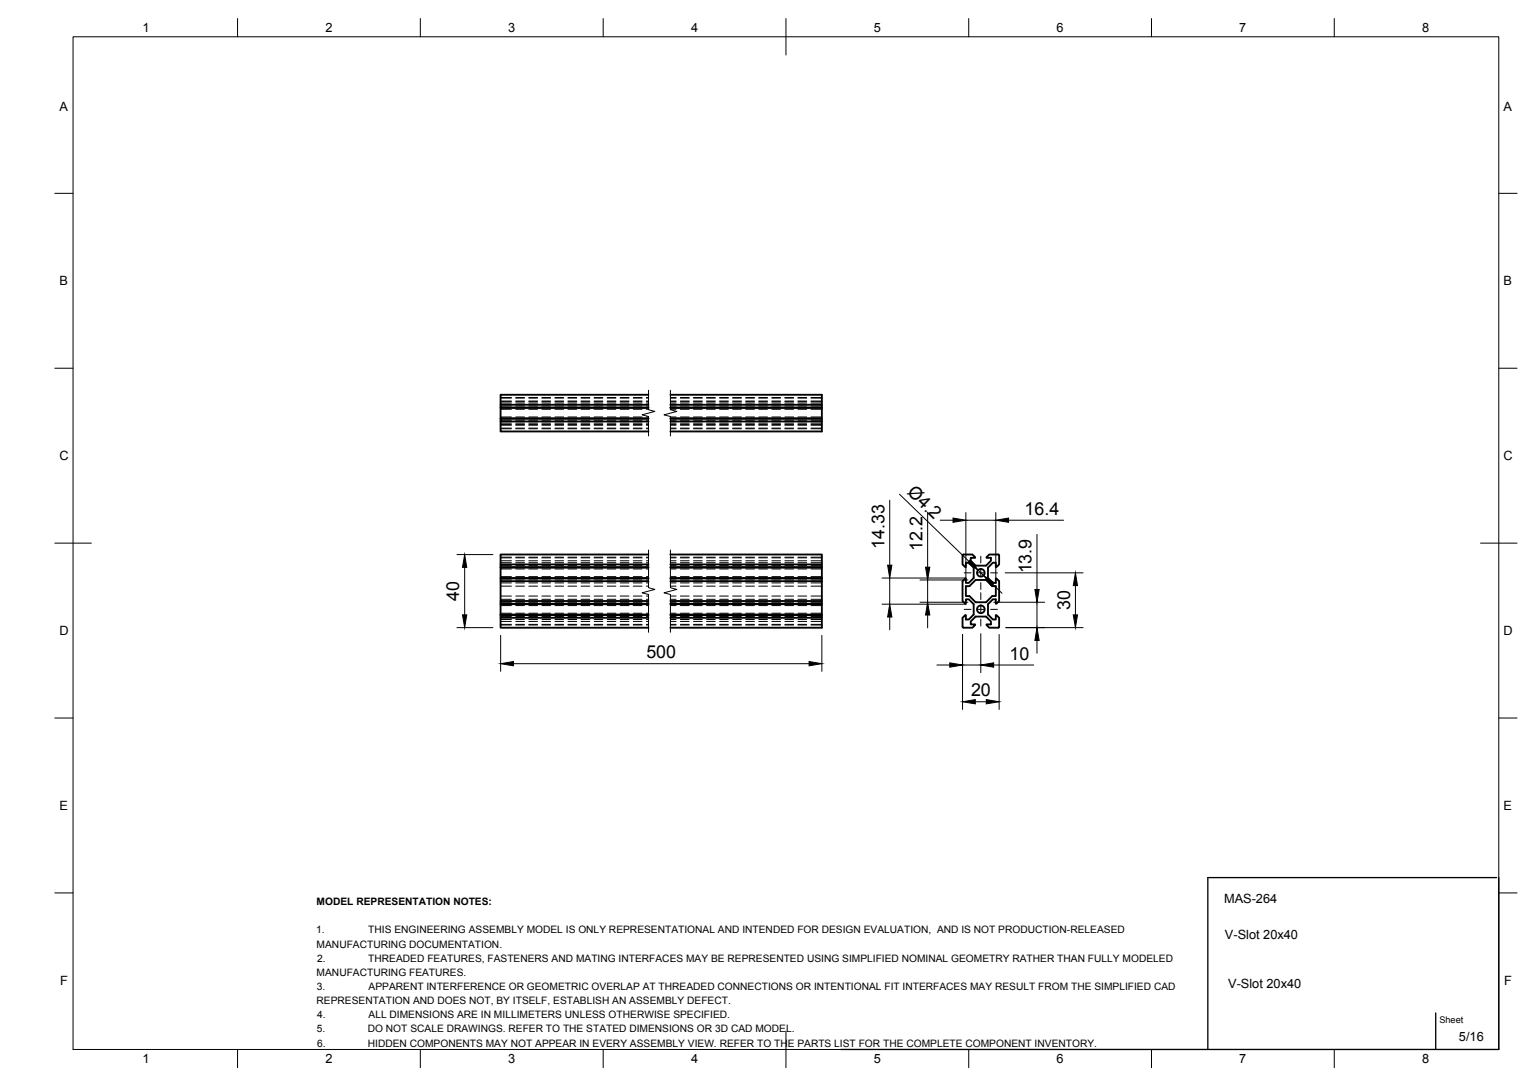
ISO-10303-21;
HEADER;
/* Generated by software containing ST-Developer
 * from STEP Tools, Inc. (www.steptools.com) 
 */

FILE_DESCRIPTION(
/* description */ (''),
/* implementation_level */ '2;1');

FILE_NAME(
/* name */ 'V-Slot 20x40.step',
/* time_stamp */ '2026-10-12T15:37:13-07:00',
/* author */ (''),
/* organization */ (''),
/* preprocessor_version */ 'ST-DEVELOPER v20.2',
/* originating_system */ 'Autodesk Translation Framework v15.15.0.0',
/* authorisation */ '');

FILE_SCHEMA (('AUTOMOTIVE_DESIGN { 1 0 10303 214 3 1 1 }'));
ENDSEC;

DATA;
#10=MECHANICAL_DESIGN_GEOMETRIC_PRESENTATION_REPRESENTATION('',(#350),#36460);
#111=SHAPE_REPRESENTATION_RELATIONSHIP('SRR','None',#36523,#124);
#124=ADVANCED_BREP_SHAPE_REPRESENTATION('',(#382),#36452);
#172=FACE_BOUND('',#2091,.T.);
#173=FACE_BOUND('',#2092,.T.);
#174=FACE_BOUND('',#2093,.T.);
#175=FACE_BOUND('',#2142,.T.);
#176=FACE_BOUND('',#2143,.T.);
#177=FACE_BOUND('',#2144,.T.);
#350=STYLED_ITEM('',(#36598),#382);
#382=MANIFOLD_SOLID_BREP('Body1',#11286);
#540=PLANE('',#12010);
#541=PLANE('',#12011);
#542=PLANE('',#12012);
#543=PLANE('',#12013);
#544=PLANE('',#12014);
#545=PLANE('',#12018);
#546=PLANE('',#12019);
#547=PLANE('',#12020);
#548=PLANE('',#12021);
#549=PLANE('',#12022);
#550=PLANE('',#12023);
#551=PLANE('',#12024);
#552=PLANE('',#12025);
#553=PLANE('',#12026);
#554=PLANE('',#12030);
#555=PLANE('',#12031);
#556=PLANE('',#12032);
#557=PLANE('',#12033);
#558=PLANE('',#12034);
#559=PLANE('',#12035);
#560=PLANE('',#12036);
#561=PLANE('',#12037);
#562=PLANE('',#12038);
#563=PLANE('',#12039);
#564=PLANE('',#12040);
#565=PLANE('',#12041);
#566=PLANE('',#12042);
#567=PLANE('',#12043);
#568=PLANE('',#12044);
#569=PLANE('',#12045);
#570=PLANE('',#12046);
#571=PLANE('',#12047);
#572=PLANE('',#12051);
#573=PLANE('',#12052);
#574=PLANE('',#12053);
#575=PLANE('',#12054);
#576=PLANE('',#12055);
#577=PLANE('',#12056);
#578=PLANE('',#12057);
#579=PLANE('',#12058);
#580=PLANE('',#12059);
#581=PLANE('',#12060);
#582=PLANE('',#12061);
#583=PLANE('',#12062);
#584=PLANE('',#12063);
#585=PLANE('',#12067);
#586=PLANE('',#12068);
#587=PLANE('',#12069);
#588=PLANE('',#12070);
#589=PLANE('',#12071);
#590=PLANE('',#12074);
#591=PLANE('',#12075);
#592=PLANE('',#12076);
#593=PLANE('',#12077);
#594=PLANE('',#12078);
#595=PLANE('',#12079);
#596=PLANE('',#12080);
#597=PLANE('',#12081);
#598=PLANE('',#12082);
#599=PLANE('',#12085);
#600=PLANE('',#12086);
#601=PLANE('',#12087);
#602=PLANE('',#12088);
#603=PLANE('',#12089);
#604=PLANE('',#12090);
#605=PLANE('',#12091);
#606=PLANE('',#12092);
#607=PLANE('',#12093);
#608=PLANE('',#12094);
#609=PLANE('',#12095);
#610=PLANE('',#12096);
#611=PLANE('',#12097);
#612=PLANE('',#12098);
#613=PLANE('',#12099);
#614=PLANE('',#12100);
#615=PLANE('',#12101);
#616=PLANE('',#12102);
#617=PLANE('',#12103);
#618=PLANE('',#12106);
#619=PLANE('',#12107);
#620=PLANE('',#12108);
#621=PLANE('',#12109);
#622=PLANE('',#12110);
#623=PLANE('',#12111);
#624=PLANE('',#12112);
#625=PLANE('',#12113);
#626=PLANE('',#12114);
#627=PLANE('',#12115);
#628=PLANE('',#12116);
#629=PLANE('',#12117);
#1389=FACE_OUTER_BOUND('',#2043,.T.);
#1390=FACE_OUTER_BOUND('',#2044,.T.);
#1391=FACE_OUTER_BOUND('',#2045,.T.);
#1392=FACE_OUTER_BOUND('',#2046,.T.);
#1393=FACE_OUTER_BOUND('',#2047,.T.);
#1394=FACE_OUTER_BOUND('',#2048,.T.);
#1395=FACE_OUTER_BOUND('',#2049,.T.);
#1396=FACE_OUTER_BOUND('',#2050,.T.);
#1397=FACE_OUTER_BOUND('',#2051,.T.);
#1398=FACE_OUTER_BOUND('',#2052,.T.);
#1399=FACE_OUTER_BOUND('',#2053,.T.);
#1400=FACE_OUTER_BOUND('',#2054,.T.);
#1401=FACE_OUTER_BOUND('',#2055,.T.);
#1402=FACE_OUTER_BOUND('',#2056,.T.);
#1403=FACE_OUTER_BOUND('',#2057,.T.);
#1404=FACE_OUTER_BOUND('',#2058,.T.);
#1405=FACE_OUTER_BOUND('',#2059,.T.);
#1406=FACE_OUTER_BOUND('',#2060,.T.);
#1407=FACE_OUTER_BOUND('',#2061,.T.);
#1408=FACE_OUTER_BOUND('',#2062,.T.);
#1409=FACE_OUTER_BOUND('',#2063,.T.);
#1410=FACE_OUTER_BOUND('',#2064,.T.);
#1411=FACE_OUTER_BOUND('',#2065,.T.);
#1412=FACE_OUTER_BOUND('',#2066,.T.);
#1413=FACE_OUTER_BOUND('',#2067,.T.);
#1414=FACE_OUTER_BOUND('',#2068,.T.);
#1415=FACE_OUTER_BOUND('',#2069,.T.);
#1416=FACE_OUTER_BOUND('',#2070,.T.);
#1417=FACE_OUTER_BOUND('',#2071,.T.);
#1418=FACE_OUTER_BOUND('',#2072,.T.);
#1419=FACE_OUTER_BOUND('',#2073,.T.);
#1420=FACE_OUTER_BOUND('',#2074,.T.);
#1421=FACE_OUTER_BOUND('',#2075,.T.);
#1422=FACE_OUTER_BOUND('',#2076,.T.);
#1423=FACE_OUTER_BOUND('',#2077,.T.);
#1424=FACE_OUTER_BOUND('',#2078,.T.);
#1425=FACE_OUTER_BOUND('',#2079,.T.);
#1426=FACE_OUTER_BOUND('',#2080,.T.);
#1427=FACE_OUTER_BOUND('',#2081,.T.);
#1428=FACE_OUTER_BOUND('',#2082,.T.);
#1429=FACE_OUTER_BOUND('',#2083,.T.);
#1430=FACE_OUTER_BOUND('',#2084,.T.);
#1431=FACE_OUTER_BOUND('',#2085,.T.);
#1432=FACE_OUTER_BOUND('',#2086,.T.);
#1433=FACE_OUTER_BOUND('',#2087,.T.);
#1434=FACE_OUTER_BOUND('',#2088,.T.);
#1435=FACE_OUTER_BOUND('',#2089,.T.);
#1436=FACE_OUTER_BOUND('',#2090,.T.);
#1437=FACE_OUTER_BOUND('',#2094,.T.);
#1438=FACE_OUTER_BOUND('',#2095,.T.);
#1439=FACE_OUTER_BOUND('',#2096,.T.);
#1440=FACE_OUTER_BOUND('',#2097,.T.);
#1441=FACE_OUTER_BOUND('',#2098,.T.);
#1442=FACE_OUTER_BOUND('',#2099,.T.);
#1443=FACE_OUTER_BOUND('',#2100,.T.);
#1444=FACE_OUTER_BOUND('',#2101,.T.);
#1445=FACE_OUTER_BOUND('',#2102,.T.);
#1446=FACE_OUTER_BOUND('',#2103,.T.);
#1447=FACE_OUTER_BOUND('',#2104,.T.);
#1448=FACE_OUTER_BOUND('',#2105,.T.);
#1449=FACE_OUTER_BOUND('',#2106,.T.);
#1450=FACE_OUTER_BOUND('',#2107,.T.);
#1451=FACE_OUTER_BOUND('',#2108,.T.);
#1452=FACE_OUTER_BOUND('',#2109,.T.);
#1453=FACE_OUTER_BOUND('',#2110,.T.);
#1454=FACE_OUTER_BOUND('',#2111,.T.);
#1455=FACE_OUTER_BOUND('',#2112,.T.);
#1456=FACE_OUTER_BOUND('',#2113,.T.);
#1457=FACE_OUTER_BOUND('',#2114,.T.);
#1458=FACE_OUTER_BOUND('',#2115,.T.);
#1459=FACE_OUTER_BOUND('',#2116,.T.);
#1460=FACE_OUTER_BOUND('',#2117,.T.);
#1461=FACE_OUTER_BOUND('',#2118,.T.);
#1462=FACE_OUTER_BOUND('',#2119,.T.);
#1463=FACE_OUTER_BOUND('',#2120,.T.);
#1464=FACE_OUTER_BOUND('',#2121,.T.);
#1465=FACE_OUTER_BOUND('',#2122,.T.);
#1466=FACE_OUTER_BOUND('',#2123,.T.);
#1467=FACE_OUTER_BOUND('',#2124,.T.);
#1468=FACE_OUTER_BOUND('',#2125,.T.);
#1469=FACE_OUTER_BOUND('',#2126,.T.);
#1470=FACE_OUTER_BOUND('',#2127,.T.);
#1471=FACE_OUTER_BOUND('',#2128,.T.);
#1472=FACE_OUTER_BOUND('',#2129,.T.);
#1473=FACE_OUTER_BOUND('',#2130,.T.);
#1474=FACE_OUTER_BOUND('',#2131,.T.);
#1475=FACE_OUTER_BOUND('',#2132,.T.);
#1476=FACE_OUTER_BOUND('',#2133,.T.);
#1477=FACE_OUTER_BOUND('',#2134,.T.);
#1478=FACE_OUTER_BOUND('',#2135,.T.);
#1479=FACE_OUTER_BOUND('',#2136,.T.);
#1480=FACE_OUTER_BOUND('',#2137,.T.);
#1481=FACE_OUTER_BOUND('',#2138,.T.);
#1482=FACE_OUTER_BOUND('',#2139,.T.);
#1483=FACE_OUTER_BOUND('',#2140,.T.);
#1484=FACE_OUTER_BOUND('',#2141,.T.);
#2043=EDGE_LOOP('',(#9050,#9051,#9052,#9053));
#2044=EDGE_LOOP('',(#9054,#9055,#9056,#9057));
#2045=EDGE_LOOP('',(#9058,#9059,#9060,#9061));
#2046=EDGE_LOOP('',(#9062,#9063,#9064,#9065));
#2047=EDGE_LOOP('',(#9066,#9067,#9068,#9069));
#2048=EDGE_LOOP('',(#9070,#9071,#9072,#9073));
#2049=EDGE_LOOP('',(#9074,#9075,#9076,#9077));
#2050=EDGE_LOOP('',(#9078,#9079,#9080,#9081));
#2051=EDGE_LOOP('',(#9082,#9083,#9084,#9085));
#2052=EDGE_LOOP('',(#9086,#9087,#9088,#9089));
#2053=EDGE_LOOP('',(#9090,#9091,#9092,#9093));
#2054=EDGE_LOOP('',(#9094,#9095,#9096,#9097));
#2055=EDGE_LOOP('',(#9098,#9099,#9100,#9101));
#2056=EDGE_LOOP('',(#9102,#9103,#9104,#9105));
#2057=EDGE_LOOP('',(#9106,#9107,#9108,#9109));
#2058=EDGE_LOOP('',(#9110,#9111,#9112,#9113));
#2059=EDGE_LOOP('',(#9114,#9115,#9116,#9117));
#2060=EDGE_LOOP('',(#9118,#9119,#9120,#9121));
#2061=EDGE_LOOP('',(#9122,#9123,#9124,#9125));
#2062=EDGE_LOOP('',(#9126,#9127,#9128,#9129));
#2063=EDGE_LOOP('',(#9130,#9131,#9132,#9133));
#2064=EDGE_LOOP('',(#9134,#9135,#9136,#9137));
#2065=EDGE_LOOP('',(#9138,#9139,#9140,#9141));
#2066=EDGE_LOOP('',(#9142,#9143,#9144,#9145));
#2067=EDGE_LOOP('',(#9146,#9147,#9148,#9149));
#2068=EDGE_LOOP('',(#9150,#9151,#9152,#9153));
#2069=EDGE_LOOP('',(#9154,#9155,#9156,#9157));
#2070=EDGE_LOOP('',(#9158,#9159,#9160,#9161));
#2071=EDGE_LOOP('',(#9162,#9163,#9164,#9165));
#2072=EDGE_LOOP('',(#9166,#9167,#9168,#9169));
#2073=EDGE_LOOP('',(#9170,#9171,#9172,#9173));
#2074=EDGE_LOOP('',(#9174,#9175,#9176,#9177));
#2075=EDGE_LOOP('',(#9178,#9179,#9180,#9181));
#2076=EDGE_LOOP('',(#9182,#9183,#9184,#9185));
#2077=EDGE_LOOP('',(#9186,#9187,#9188,#9189));
#2078=EDGE_LOOP('',(#9190,#9191,#9192,#9193));
#2079=EDGE_LOOP('',(#9194,#9195,#9196,#9197));
#2080=EDGE_LOOP('',(#9198,#9199,#9200,#9201));
#2081=EDGE_LOOP('',(#9202,#9203,#9204,#9205));
#2082=EDGE_LOOP('',(#9206,#9207,#9208,#9209));
#2083=EDGE_LOOP('',(#9210,#9211,#9212,#9213));
#2084=EDGE_LOOP('',(#9214,#9215,#9216,#9217));
#2085=EDGE_LOOP('',(#9218,#9219,#9220,#9221));
#2086=EDGE_LOOP('',(#9222,#9223,#9224,#9225));
#2087=EDGE_LOOP('',(#9226,#9227,#9228,#9229));
#2088=EDGE_LOOP('',(#9230,#9231,#9232,#9233));
#2089=EDGE_LOOP('',(#9234,#9235,#9236,#9237));
#2090=EDGE_LOOP('',(#9238,#9239,#9240,#9241,#9242,#9243,#9244,#9245,#9246,
#9247,#9248,#9249,#9250,#9251,#9252,#9253,#9254,#9255,#9256,#9257,#9258,
#9259,#9260,#9261,#9262,#9263,#9264,#9265,#9266,#9267,#9268,#9269,#9270,
#9271,#9272,#9273,#9274,#9275,#9276,#9277,#9278,#9279,#9280,#9281,#9282,
#9283,#9284,#9285,#9286,#9287,#9288,#9289,#9290,#9291,#9292,#9293,#9294,
#9295,#9296,#9297,#9298,#9299,#9300,#9301,#9302,#9303,#9304,#9305,#9306,
#9307,#9308,#9309,#9310,#9311,#9312,#9313,#9314,#9315,#9316,#9317));
#2091=EDGE_LOOP('',(#9318,#9319,#9320,#9321,#9322,#9323,#9324,#9325,#9326,
#9327,#9328,#9329));
#2092=EDGE_LOOP('',(#9330));
#2093=EDGE_LOOP('',(#9331));
#2094=EDGE_LOOP('',(#9332,#9333,#9334,#9335));
#2095=EDGE_LOOP('',(#9336,#9337,#9338,#9339));
#2096=EDGE_LOOP('',(#9340,#9341,#9342,#9343));
#2097=EDGE_LOOP('',(#9344,#9345,#9346,#9347));
#2098=EDGE_LOOP('',(#9348,#9349,#9350,#9351));
#2099=EDGE_LOOP('',(#9352,#9353,#9354,#9355));
#2100=EDGE_LOOP('',(#9356,#9357,#9358,#9359));
#2101=EDGE_LOOP('',(#9360,#9361,#9362,#9363));
#2102=EDGE_LOOP('',(#9364,#9365,#9366,#9367));
#2103=EDGE_LOOP('',(#9368,#9369,#9370,#9371));
#2104=EDGE_LOOP('',(#9372,#9373,#9374,#9375));
#2105=EDGE_LOOP('',(#9376,#9377,#9378,#9379));
#2106=EDGE_LOOP('',(#9380,#9381,#9382,#9383));
#2107=EDGE_LOOP('',(#9384,#9385,#9386,#9387));
#2108=EDGE_LOOP('',(#9388,#9389,#9390,#9391));
#2109=EDGE_LOOP('',(#9392,#9393,#9394,#9395));
#2110=EDGE_LOOP('',(#9396,#9397,#9398,#9399));
#2111=EDGE_LOOP('',(#9400,#9401,#9402,#9403));
#2112=EDGE_LOOP('',(#9404,#9405,#9406,#9407));
#2113=EDGE_LOOP('',(#9408,#9409,#9410,#9411));
#2114=EDGE_LOOP('',(#9412,#9413,#9414,#9415));
#2115=EDGE_LOOP('',(#9416,#9417,#9418,#9419));
#2116=EDGE_LOOP('',(#9420,#9421,#9422,#9423));
#2117=EDGE_LOOP('',(#9424,#9425,#9426,#9427));
#2118=EDGE_LOOP('',(#9428,#9429,#9430,#9431));
#2119=EDGE_LOOP('',(#9432,#9433,#9434,#9435));
#2120=EDGE_LOOP('',(#9436,#9437,#9438,#9439));
#2121=EDGE_LOOP('',(#9440,#9441,#9442,#9443));
#2122=EDGE_LOOP('',(#9444,#9445,#9446,#9447));
#2123=EDGE_LOOP('',(#9448,#9449,#9450,#9451));
#2124=EDGE_LOOP('',(#9452,#9453,#9454,#9455));
#2125=EDGE_LOOP('',(#9456,#9457,#9458,#9459));
#2126=EDGE_LOOP('',(#9460,#9461,#9462,#9463));
#2127=EDGE_LOOP('',(#9464,#9465,#9466,#9467));
#2128=EDGE_LOOP('',(#9468,#9469,#9470,#9471));
#2129=EDGE_LOOP('',(#9472,#9473,#9474,#9475));
#2130=EDGE_LOOP('',(#9476,#9477,#9478,#9479));
#2131=EDGE_LOOP('',(#9480,#9481,#9482,#9483));
#2132=EDGE_LOOP('',(#9484,#9485,#9486,#9487));
#2133=EDGE_LOOP('',(#9488,#9489,#9490,#9491));
#2134=EDGE_LOOP('',(#9492,#9493,#9494,#9495));
#2135=EDGE_LOOP('',(#9496,#9497,#9498,#9499));
#2136=EDGE_LOOP('',(#9500,#9501,#9502,#9503));
#2137=EDGE_LOOP('',(#9504,#9505,#9506,#9507));
#2138=EDGE_LOOP('',(#9508,#9509,#9510,#9511));
#2139=EDGE_LOOP('',(#9512,#9513,#9514,#9515));
#2140=EDGE_LOOP('',(#9516,#9517,#9518,#9519));
#2141=EDGE_LOOP('',(#9520,#9521,#9522,#9523,#9524,#9525,#9526,#9527,#9528,
#9529,#9530,#9531,#9532,#9533,#9534,#9535,#9536,#9537,#9538,#9539,#9540,
#9541,#9542,#9543,#9544,#9545,#9546,#9547,#9548,#9549,#9550,#9551,#9552,
#9553,#9554,#9555,#9556,#9557,#9558,#9559,#9560,#9561,#9562,#9563,#9564,
#9565,#9566,#9567,#9568,#9569,#9570,#9571,#9572,#9573,#9574,#9575,#9576,
#9577,#9578,#9579,#9580,#9581,#9582,#9583,#9584,#9585,#9586,#9587,#9588,
#9589,#9590,#9591,#9592,#9593,#9594,#9595,#9596,#9597,#9598,#9599));
#2142=EDGE_LOOP('',(#9600));
#2143=EDGE_LOOP('',(#9601,#9602,#9603,#9604,#9605,#9606,#9607,#9608,#9609,
#9610,#9611,#9612));
#2144=EDGE_LOOP('',(#9613));
#2812=LINE('',#34888,#3758);
#2813=LINE('',#34890,#3759);
#2814=LINE('',#34892,#3760);
#2815=LINE('',#34893,#3761);
#2816=LINE('',#34897,#3762);
#2817=LINE('',#34899,#3763);
#2818=LINE('',#34901,#3764);
#2819=LINE('',#34902,#3765);
#2820=LINE('',#34906,#3766);
#2821=LINE('',#34908,#3767);
#2822=LINE('',#34910,#3768);
#2823=LINE('',#34911,#3769);
#2824=LINE('',#34915,#3770);
#2825=LINE('',#34917,#3771);
#2826=LINE('',#34919,#3772);
#2827=LINE('',#34920,#3773);
#2828=LINE('',#34924,#3774);
#2829=LINE('',#34926,#3775);
#2830=LINE('',#34928,#3776);
#2831=LINE('',#34929,#3777);
#2832=LINE('',#34934,#3778);
#2833=LINE('',#34939,#3779);
#2834=LINE('',#34941,#3780);
#2835=LINE('',#34943,#3781);
#2836=LINE('',#34944,#3782);
#2837=LINE('',#34948,#3783);
#2838=LINE('',#34950,#3784);
#2839=LINE('',#34952,#3785);
#2840=LINE('',#34953,#3786);
#2841=LINE('',#34955,#3787);
#2842=LINE('',#34956,#3788);
#2843=LINE('',#34959,#3789);
#2844=LINE('',#34961,#3790);
#2845=LINE('',#34962,#3791);
#2846=LINE('',#34965,#3792);
#2847=LINE('',#34967,#3793);
#2848=LINE('',#34968,#3794);
#2849=LINE('',#34971,#3795);
#2850=LINE('',#34973,#3796);
#2851=LINE('',#34974,#3797);
#2852=LINE('',#34977,#3798);
#2853=LINE('',#34979,#3799);
#2854=LINE('',#34980,#3800);
#2855=LINE('',#34983,#3801);
#2856=LINE('',#34985,#3802);
#2857=LINE('',#34986,#3803);
#2858=LINE('',#34989,#3804);
#2859=LINE('',#34991,#3805);
#2860=LINE('',#34992,#3806);
#2861=LINE('',#34997,#3807);
#2862=LINE('',#35001,#3808);
#2863=LINE('',#35003,#3809);
#2864=LINE('',#35004,#3810);
#2865=LINE('',#35007,#3811);
#2866=LINE('',#35009,#3812);
#2867=LINE('',#35010,#3813);
#2868=LINE('',#35013,#3814);
#2869=LINE('',#35015,#3815);
#2870=LINE('',#35016,#3816);
#2871=LINE('',#35018,#3817);
#2872=LINE('',#35019,#3818);
#2873=LINE('',#35023,#3819);
#2874=LINE('',#35025,#3820);
#2875=LINE('',#35027,#3821);
#2876=LINE('',#35028,#3822);
#2877=LINE('',#35030,#3823);
#2878=LINE('',#35031,#3824);
#2879=LINE('',#35033,#3825);
#2880=LINE('',#35034,#3826);
#2881=LINE('',#35038,#3827);
#2882=LINE('',#35040,#3828);
#2883=LINE('',#35042,#3829);
#2884=LINE('',#35043,#3830);
#2885=LINE('',#35046,#3831);
#2886=LINE('',#35048,#3832);
#2887=LINE('',#35049,#3833);
#2888=LINE('',#35051,#3834);
#2889=LINE('',#35052,#3835);
#2890=LINE('',#35056,#3836);
#2891=LINE('',#35058,#3837);
#2892=LINE('',#35060,#3838);
#2893=LINE('',#35061,#3839);
#2894=LINE('',#35063,#3840);
#2895=LINE('',#35064,#3841);
#2896=LINE('',#35067,#3842);
#2897=LINE('',#35069,#3843);
#2898=LINE('',#35070,#3844);
#2899=LINE('',#35073,#3845);
#2900=LINE('',#35075,#3846);
#2901=LINE('',#35076,#3847);
#2902=LINE('',#35079,#3848);
#2903=LINE('',#35081,#3849);
#2904=LINE('',#35082,#3850);
#2905=LINE('',#35085,#3851);
#2906=LINE('',#35087,#3852);
#2907=LINE('',#35088,#3853);
#2908=LINE('',#35091,#3854);
#2909=LINE('',#35093,#3855);
#2910=LINE('',#35094,#3856);
#2911=LINE('',#35097,#3857);
#2912=LINE('',#35099,#3858);
#2913=LINE('',#35100,#3859);
#2914=LINE('',#35105,#3860);
#2915=LINE('',#35109,#3861);
#2916=LINE('',#35111,#3862);
#2917=LINE('',#35112,#3863);
#2918=LINE('',#35115,#3864);
#2919=LINE('',#35117,#3865);
#2920=LINE('',#35118,#3866);
#2921=LINE('',#35121,#3867);
#2922=LINE('',#35123,#3868);
#2923=LINE('',#35124,#3869);
#2924=LINE('',#35126,#3870);
#2925=LINE('',#35127,#3871);
#2926=LINE('',#35129,#3872);
#2927=LINE('',#35130,#3873);
#2928=LINE('',#35133,#3874);
#2929=LINE('',#35135,#3875);
#2930=LINE('',#35136,#3876);
#2931=LINE('',#35139,#3877);
#2932=LINE('',#35141,#3878);
#2933=LINE('',#35142,#3879);
#2934=LINE('',#35145,#3880);
#2935=LINE('',#35147,#3881);
#2936=LINE('',#35148,#3882);
#2937=LINE('',#35151,#3883);
#2938=LINE('',#35153,#3884);
#2939=LINE('',#35154,#3885);
#2940=LINE('',#35157,#3886);
#2941=LINE('',#35159,#3887);
#2942=LINE('',#35160,#3888);
#2943=LINE('',#35163,#3889);
#2944=LINE('',#35165,#3890);
#2945=LINE('',#35166,#3891);
#2946=LINE('',#35169,#3892);
#2947=LINE('',#35171,#3893);
#2948=LINE('',#35172,#3894);
#2949=LINE('',#35175,#3895);
#2950=LINE('',#35177,#3896);
#2951=LINE('',#35179,#3897);
#2952=LINE('',#35181,#3898);
#2953=LINE('',#35183,#3899);
#2954=LINE('',#35185,#3900);
#2955=LINE('',#35187,#3901);
#2956=LINE('',#35189,#3902);
#2957=LINE('',#35191,#3903);
#2958=LINE('',#35193,#3904);
#2959=LINE('',#35195,#3905);
#2960=LINE('',#35197,#3906);
#2961=LINE('',#35199,#3907);
#2962=LINE('',#35201,#3908);
#2963=LINE('',#35205,#3909);
#2964=LINE('',#35207,#3910);
#2965=LINE('',#35209,#3911);
#2966=LINE('',#35211,#3912);
#2967=LINE('',#35213,#3913);
#2968=LINE('',#35215,#3914);
#2969=LINE('',#35217,#3915);
#2970=LINE('',#35219,#3916);
#2971=LINE('',#35221,#3917);
#2972=LINE('',#35223,#3918);
#2973=LINE('',#35225,#3919);
#2974=LINE('',#35227,#3920);
#2975=LINE('',#35229,#3921);
#2976=LINE('',#35233,#3922);
#2977=LINE('',#35235,#3923);
#2978=LINE('',#35237,#3924);
#2979=LINE('',#35239,#3925);
#2980=LINE('',#35241,#3926);
#2981=LINE('',#35243,#3927);
#2982=LINE('',#35245,#3928);
#2983=LINE('',#35247,#3929);
#2984=LINE('',#35249,#3930);
#2985=LINE('',#35251,#3931);
#2986=LINE('',#35253,#3932);
#2987=LINE('',#35254,#3933);
#2988=LINE('',#35256,#3934);
#2989=LINE('',#35258,#3935);
#2990=LINE('',#35260,#3936);
#2991=LINE('',#35262,#3937);
#2992=LINE('',#35263,#3938);
#2993=LINE('',#35268,#3939);
#2994=LINE('',#35269,#3940);
#2995=LINE('',#35272,#3941);
#2996=LINE('',#35273,#3942);
#2997=LINE('',#35276,#3943);
#2998=LINE('',#35278,#3944);
#2999=LINE('',#35279,#3945);
#3000=LINE('',#35282,#3946);
#3001=LINE('',#35284,#3947);
#3002=LINE('',#35285,#3948);
#3003=LINE('',#35288,#3949);
#3004=LINE('',#35290,#3950);
#3005=LINE('',#35291,#3951);
#3006=LINE('',#35294,#3952);
#3007=LINE('',#35298,#3953);
#3008=LINE('',#35300,#3954);
#3009=LINE('',#35301,#3955);
#3010=LINE('',#35304,#3956);
#3011=LINE('',#35306,#3957);
#3012=LINE('',#35307,#3958);
#3013=LINE('',#35309,#3959);
#3014=LINE('',#35312,#3960);
#3015=LINE('',#35313,#3961);
#3016=LINE('',#35316,#3962);
#3017=LINE('',#35317,#3963);
#3018=LINE('',#35320,#3964);
#3019=LINE('',#35321,#3965);
#3020=LINE('',#35324,#3966);
#3021=LINE('',#35325,#3967);
#3022=LINE('',#35328,#3968);
#3023=LINE('',#35329,#3969);
#3024=LINE('',#35332,#3970);
#3025=LINE('',#35333,#3971);
#3026=LINE('',#35337,#3972);
#3027=LINE('',#35340,#3973);
#3028=LINE('',#35341,#3974);
#3029=LINE('',#35344,#3975);
#3030=LINE('',#35345,#3976);
#3031=LINE('',#35348,#3977);
#3032=LINE('',#35349,#3978);
#3033=LINE('',#35351,#3979);
#3034=LINE('',#35354,#3980);
#3035=LINE('',#35356,#3981);
#3036=LINE('',#35357,#3982);
#3037=LINE('',#35359,#3983);
#3038=LINE('',#35361,#3984);
#3039=LINE('',#35364,#3985);
#3040=LINE('',#35365,#3986);
#3041=LINE('',#35368,#3987);
#3042=LINE('',#35369,#3988);
#3043=LINE('',#35372,#3989);
#3044=LINE('',#35373,#3990);
#3045=LINE('',#35375,#3991);
#3046=LINE('',#35378,#3992);
#3047=LINE('',#35380,#3993);
#3048=LINE('',#35381,#3994);
#3049=LINE('',#35383,#3995);
#3050=LINE('',#35386,#3996);
#3051=LINE('',#35387,#3997);
#3052=LINE('',#35390,#3998);
#3053=LINE('',#35391,#3999);
#3054=LINE('',#35394,#4000);
#3055=LINE('',#35395,#4001);
#3056=LINE('',#35398,#4002);
#3057=LINE('',#35399,#4003);
#3058=LINE('',#35402,#4004);
#3059=LINE('',#35403,#4005);
#3060=LINE('',#35406,#4006);
#3061=LINE('',#35407,#4007);
#3062=LINE('',#35411,#4008);
#3063=LINE('',#35414,#4009);
#3064=LINE('',#35415,#4010);
#3065=LINE('',#35418,#4011);
#3066=LINE('',#35419,#4012);
#3067=LINE('',#35422,#4013);
#3068=LINE('',#35423,#4014);
#3069=LINE('',#35425,#4015);
#3070=LINE('',#35427,#4016);
#3071=LINE('',#35430,#4017);
#3072=LINE('',#35431,#4018);
#3073=LINE('',#35434,#4019);
#3074=LINE('',#35435,#4020);
#3075=LINE('',#35438,#4021);
#3076=LINE('',#35439,#4022);
#3077=LINE('',#35442,#4023);
#3078=LINE('',#35443,#4024);
#3079=LINE('',#35446,#4025);
#3080=LINE('',#35447,#4026);
#3081=LINE('',#35449,#4027);
#3758=VECTOR('',#14007,10.);
#3759=VECTOR('',#14008,10.);
#3760=VECTOR('',#14009,10.);
#3761=VECTOR('',#14010,10.);
#3762=VECTOR('',#14013,10.);
#3763=VECTOR('',#14014,10.);
#3764=VECTOR('',#14015,10.);
#3765=VECTOR('',#14016,10.);
#3766=VECTOR('',#14019,10.);
#3767=VECTOR('',#14020,10.);
#3768=VECTOR('',#14021,10.);
#3769=VECTOR('',#14022,10.);
#3770=VECTOR('',#14025,10.);
#3771=VECTOR('',#14026,10.);
#3772=VECTOR('',#14027,10.);
#3773=VECTOR('',#14028,10.);
#3774=VECTOR('',#14031,10.);
#3775=VECTOR('',#14032,10.);
#3776=VECTOR('',#14033,10.);
#3777=VECTOR('',#14034,10.);
#3778=VECTOR('',#14039,2.1);
#3779=VECTOR('',#14044,10.);
#3780=VECTOR('',#14045,10.);
#3781=VECTOR('',#14046,10.);
#3782=VECTOR('',#14047,10.);
#3783=VECTOR('',#14050,10.);
#3784=VECTOR('',#14051,10.);
#3785=VECTOR('',#14052,10.);
#3786=VECTOR('',#14053,10.);
#3787=VECTOR('',#14056,10.);
#3788=VECTOR('',#14057,10.);
#3789=VECTOR('',#14060,10.);
#3790=VECTOR('',#14061,10.);
#3791=VECTOR('',#14062,10.);
#3792=VECTOR('',#14065,10.);
#3793=VECTOR('',#14066,10.);
#3794=VECTOR('',#14067,10.);
#3795=VECTOR('',#14070,10.);
#3796=VECTOR('',#14071,10.);
#3797=VECTOR('',#14072,10.);
#3798=VECTOR('',#14075,10.);
#3799=VECTOR('',#14076,10.);
#3800=VECTOR('',#14077,10.);
#3801=VECTOR('',#14080,10.);
#3802=VECTOR('',#14081,10.);
#3803=VECTOR('',#14082,10.);
#3804=VECTOR('',#14085,10.);
#3805=VECTOR('',#14086,10.);
#3806=VECTOR('',#14087,10.);
#3807=VECTOR('',#14092,10.);
#3808=VECTOR('',#14097,10.);
#3809=VECTOR('',#14098,10.);
#3810=VECTOR('',#14099,10.);
#3811=VECTOR('',#14102,10.);
#3812=VECTOR('',#14103,10.);
#3813=VECTOR('',#14104,10.);
#3814=VECTOR('',#14107,10.);
#3815=VECTOR('',#14108,10.);
#3816=VECTOR('',#14109,10.);
#3817=VECTOR('',#14112,10.);
#3818=VECTOR('',#14113,10.);
#3819=VECTOR('',#14116,10.);
#3820=VECTOR('',#14117,10.);
#3821=VECTOR('',#14118,10.);
#3822=VECTOR('',#14119,10.);
#3823=VECTOR('',#14122,10.);
#3824=VECTOR('',#14123,10.);
#3825=VECTOR('',#14126,10.);
#3826=VECTOR('',#14127,10.);
#3827=VECTOR('',#14130,10.);
#3828=VECTOR('',#14131,10.);
#3829=VECTOR('',#14132,10.);
#3830=VECTOR('',#14133,10.);
#3831=VECTOR('',#14136,10.);
#3832=VECTOR('',#14137,10.);
#3833=VECTOR('',#14138,10.);
#3834=VECTOR('',#14141,10.);
#3835=VECTOR('',#14142,10.);
#3836=VECTOR('',#14145,10.);
#3837=VECTOR('',#14146,10.);
#3838=VECTOR('',#14147,10.);
#3839=VECTOR('',#14148,10.);
#3840=VECTOR('',#14151,10.);
#3841=VECTOR('',#14152,10.);
#3842=VECTOR('',#14155,10.);
#3843=VECTOR('',#14156,10.);
#3844=VECTOR('',#14157,10.);
#3845=VECTOR('',#14160,10.);
#3846=VECTOR('',#14161,10.);
#3847=VECTOR('',#14162,10.);
#3848=VECTOR('',#14165,10.);
#3849=VECTOR('',#14166,10.);
#3850=VECTOR('',#14167,10.);
#3851=VECTOR('',#14170,10.);
#3852=VECTOR('',#14171,10.);
#3853=VECTOR('',#14172,10.);
#3854=VECTOR('',#14175,10.);
#3855=VECTOR('',#14176,10.);
#3856=VECTOR('',#14177,10.);
#3857=VECTOR('',#14180,10.);
#3858=VECTOR('',#14181,10.);
#3859=VECTOR('',#14182,10.);
#3860=VECTOR('',#14187,10.);
#3861=VECTOR('',#14192,10.);
#3862=VECTOR('',#14193,10.);
#3863=VECTOR('',#14194,10.);
#3864=VECTOR('',#14197,10.);
#3865=VECTOR('',#14198,10.);
#3866=VECTOR('',#14199,10.);
#3867=VECTOR('',#14202,10.);
#3868=VECTOR('',#14203,10.);
#3869=VECTOR('',#14204,10.);
#3870=VECTOR('',#14207,10.);
#3871=VECTOR('',#14208,10.);
#3872=VECTOR('',#14211,10.);
#3873=VECTOR('',#14212,10.);
#3874=VECTOR('',#14215,10.);
#3875=VECTOR('',#14216,10.);
#3876=VECTOR('',#14217,10.);
#3877=VECTOR('',#14220,10.);
#3878=VECTOR('',#14221,10.);
#3879=VECTOR('',#14222,10.);
#3880=VECTOR('',#14225,10.);
#3881=VECTOR('',#14226,10.);
#3882=VECTOR('',#14227,10.);
#3883=VECTOR('',#14230,10.);
#3884=VECTOR('',#14231,10.);
#3885=VECTOR('',#14232,10.);
#3886=VECTOR('',#14235,10.);
#3887=VECTOR('',#14236,10.);
#3888=VECTOR('',#14237,10.);
#3889=VECTOR('',#14240,10.);
#3890=VECTOR('',#14241,10.);
#3891=VECTOR('',#14242,10.);
#3892=VECTOR('',#14245,10.);
#3893=VECTOR('',#14246,10.);
#3894=VECTOR('',#14247,10.);
#3895=VECTOR('',#14250,10.);
#3896=VECTOR('',#14251,10.);
#3897=VECTOR('',#14252,10.);
#3898=VECTOR('',#14253,10.);
#3899=VECTOR('',#14254,10.);
#3900=VECTOR('',#14255,10.);
#3901=VECTOR('',#14256,10.);
#3902=VECTOR('',#14257,10.);
#3903=VECTOR('',#14258,10.);
#3904=VECTOR('',#14259,10.);
#3905=VECTOR('',#14260,10.);
#3906=VECTOR('',#14261,10.);
#3907=VECTOR('',#14262,10.);
#3908=VECTOR('',#14263,10.);
#3909=VECTOR('',#14266,10.);
#3910=VECTOR('',#14267,10.);
#3911=VECTOR('',#14268,10.);
#3912=VECTOR('',#14269,10.);
#3913=VECTOR('',#14270,10.);
#3914=VECTOR('',#14271,10.);
#3915=VECTOR('',#14272,10.);
#3916=VECTOR('',#14273,10.);
#3917=VECTOR('',#14274,10.);
#3918=VECTOR('',#14275,10.);
#3919=VECTOR('',#14276,10.);
#3920=VECTOR('',#14277,10.);
#3921=VECTOR('',#14278,10.);
#3922=VECTOR('',#14281,10.);
#3923=VECTOR('',#14282,10.);
#3924=VECTOR('',#14283,10.);
#3925=VECTOR('',#14284,10.);
#3926=VECTOR('',#14285,10.);
#3927=VECTOR('',#14286,10.);
#3928=VECTOR('',#14287,10.);
#3929=VECTOR('',#14288,10.);
#3930=VECTOR('',#14289,10.);
#3931=VECTOR('',#14290,10.);
#3932=VECTOR('',#14291,10.);
#3933=VECTOR('',#14292,10.);
#3934=VECTOR('',#14293,10.);
#3935=VECTOR('',#14294,10.);
#3936=VECTOR('',#14295,10.);
#3937=VECTOR('',#14296,10.);
#3938=VECTOR('',#14297,10.);
#3939=VECTOR('',#14302,10.);
#3940=VECTOR('',#14303,10.);
#3941=VECTOR('',#14306,10.);
#3942=VECTOR('',#14307,10.);
#3943=VECTOR('',#14310,10.);
#3944=VECTOR('',#14311,10.);
#3945=VECTOR('',#14312,10.);
#3946=VECTOR('',#14315,10.);
#3947=VECTOR('',#14316,10.);
#3948=VECTOR('',#14317,10.);
#3949=VECTOR('',#14320,10.);
#3950=VECTOR('',#14321,10.);
#3951=VECTOR('',#14322,10.);
#3952=VECTOR('',#14325,2.1);
#3953=VECTOR('',#14330,10.);
#3954=VECTOR('',#14331,10.);
#3955=VECTOR('',#14332,10.);
#3956=VECTOR('',#14335,10.);
#3957=VECTOR('',#14336,10.);
#3958=VECTOR('',#14337,10.);
#3959=VECTOR('',#14340,10.);
#3960=VECTOR('',#14343,10.);
#3961=VECTOR('',#14344,10.);
#3962=VECTOR('',#14347,10.);
#3963=VECTOR('',#14348,10.);
#3964=VECTOR('',#14351,10.);
#3965=VECTOR('',#14352,10.);
#3966=VECTOR('',#14355,10.);
#3967=VECTOR('',#14356,10.);
#3968=VECTOR('',#14359,10.);
#3969=VECTOR('',#14360,10.);
#3970=VECTOR('',#14363,10.);
#3971=VECTOR('',#14364,10.);
#3972=VECTOR('',#14369,10.);
#3973=VECTOR('',#14372,10.);
#3974=VECTOR('',#14373,10.);
#3975=VECTOR('',#14376,10.);
#3976=VECTOR('',#14377,10.);
#3977=VECTOR('',#14380,10.);
#3978=VECTOR('',#14381,10.);
#3979=VECTOR('',#14384,10.);
#3980=VECTOR('',#14387,10.);
#3981=VECTOR('',#14388,10.);
#3982=VECTOR('',#14389,10.);
#3983=VECTOR('',#14392,10.);
#3984=VECTOR('',#14395,10.);
#3985=VECTOR('',#14398,10.);
#3986=VECTOR('',#14399,10.);
#3987=VECTOR('',#14402,10.);
#3988=VECTOR('',#14403,10.);
#3989=VECTOR('',#14406,10.);
#3990=VECTOR('',#14407,10.);
#3991=VECTOR('',#14410,10.);
#3992=VECTOR('',#14413,10.);
#3993=VECTOR('',#14414,10.);
#3994=VECTOR('',#14415,10.);
#3995=VECTOR('',#14418,10.);
#3996=VECTOR('',#14421,10.);
#3997=VECTOR('',#14422,10.);
#3998=VECTOR('',#14425,10.);
#3999=VECTOR('',#14426,10.);
#4000=VECTOR('',#14429,10.);
#4001=VECTOR('',#14430,10.);
#4002=VECTOR('',#14433,10.);
#4003=VECTOR('',#14434,10.);
#4004=VECTOR('',#14437,10.);
#4005=VECTOR('',#14438,10.);
#4006=VECTOR('',#14441,10.);
#4007=VECTOR('',#14442,10.);
#4008=VECTOR('',#14447,10.);
#4009=VECTOR('',#14450,10.);
#4010=VECTOR('',#14451,10.);
#4011=VECTOR('',#14454,10.);
#4012=VECTOR('',#14455,10.);
#4013=VECTOR('',#14458,10.);
#4014=VECTOR('',#14459,10.);
#4015=VECTOR('',#14462,10.);
#4016=VECTOR('',#14465,10.);
#4017=VECTOR('',#14468,10.);
#4018=VECTOR('',#14469,10.);
#4019=VECTOR('',#14472,10.);
#4020=VECTOR('',#14473,10.);
#4021=VECTOR('',#14476,10.);
#4022=VECTOR('',#14477,10.);
#4023=VECTOR('',#14480,10.);
#4024=VECTOR('',#14481,10.);
#4025=VECTOR('',#14484,10.);
#4026=VECTOR('',#14485,10.);
#4027=VECTOR('',#14488,10.);
#4441=CIRCLE('',#12016,2.1);
#4442=CIRCLE('',#12017,2.1);
#4443=CIRCLE('',#12028,0.500000000000003);
#4444=CIRCLE('',#12029,0.500000000000003);
#4445=CIRCLE('',#12049,0.500000000000003);
#4446=CIRCLE('',#12050,0.500000000000003);
#4447=CIRCLE('',#12064,0.500000000000003);
#4448=CIRCLE('',#12065,0.500000000000003);
#4449=CIRCLE('',#12066,2.1);
#4450=CIRCLE('',#12073,2.1);
#4451=CIRCLE('',#12084,0.500000000000003);
#4452=CIRCLE('',#12105,0.500000000000003);
#5199=VERTEX_POINT('',#34886);
#5200=VERTEX_POINT('',#34887);
#5201=VERTEX_POINT('',#34889);
#5202=VERTEX_POINT('',#34891);
#5203=VERTEX_POINT('',#34895);
#5204=VERTEX_POINT('',#34896);
#5205=VERTEX_POINT('',#34898);
#5206=VERTEX_POINT('',#34900);
#5207=VERTEX_POINT('',#34904);
#5208=VERTEX_POINT('',#34905);
#5209=VERTEX_POINT('',#34907);
#5210=VERTEX_POINT('',#34909);
#5211=VERTEX_POINT('',#34913);
#5212=VERTEX_POINT('',#34914);
#5213=VERTEX_POINT('',#34916);
#5214=VERTEX_POINT('',#34918);
#5215=VERTEX_POINT('',#34922);
#5216=VERTEX_POINT('',#34923);
#5217=VERTEX_POINT('',#34925);
#5218=VERTEX_POINT('',#34927);
#5219=VERTEX_POINT('',#34931);
#5220=VERTEX_POINT('',#34933);
#5221=VERTEX_POINT('',#34937);
#5222=VERTEX_POINT('',#34938);
#5223=VERTEX_POINT('',#34940);
#5224=VERTEX_POINT('',#34942);
#5225=VERTEX_POINT('',#34946);
#5226=VERTEX_POINT('',#34947);
#5227=VERTEX_POINT('',#34949);
#5228=VERTEX_POINT('',#34951);
#5229=VERTEX_POINT('',#34958);
#5230=VERTEX_POINT('',#34960);
#5231=VERTEX_POINT('',#34964);
#5232=VERTEX_POINT('',#34966);
#5233=VERTEX_POINT('',#34970);
#5234=VERTEX_POINT('',#34972);
#5235=VERTEX_POINT('',#34976);
#5236=VERTEX_POINT('',#34978);
#5237=VERTEX_POINT('',#34982);
#5238=VERTEX_POINT('',#34984);
#5239=VERTEX_POINT('',#34988);
#5240=VERTEX_POINT('',#34990);
#5241=VERTEX_POINT('',#34994);
#5242=VERTEX_POINT('',#34996);
#5243=VERTEX_POINT('',#35000);
#5244=VERTEX_POINT('',#35002);
#5245=VERTEX_POINT('',#35006);
#5246=VERTEX_POINT('',#35008);
#5247=VERTEX_POINT('',#35012);
#5248=VERTEX_POINT('',#35014);
#5249=VERTEX_POINT('',#35021);
#5250=VERTEX_POINT('',#35022);
#5251=VERTEX_POINT('',#35024);
#5252=VERTEX_POINT('',#35026);
#5253=VERTEX_POINT('',#35036);
#5254=VERTEX_POINT('',#35037);
#5255=VERTEX_POINT('',#35039);
#5256=VERTEX_POINT('',#35041);
#5257=VERTEX_POINT('',#35045);
#5258=VERTEX_POINT('',#35047);
#5259=VERTEX_POINT('',#35054);
#5260=VERTEX_POINT('',#35055);
#5261=VERTEX_POINT('',#35057);
#5262=VERTEX_POINT('',#35059);
#5263=VERTEX_POINT('',#35066);
#5264=VERTEX_POINT('',#35068);
#5265=VERTEX_POINT('',#35072);
#5266=VERTEX_POINT('',#35074);
#5267=VERTEX_POINT('',#35078);
#5268=VERTEX_POINT('',#35080);
#5269=VERTEX_POINT('',#35084);
#5270=VERTEX_POINT('',#35086);
#5271=VERTEX_POINT('',#35090);
#5272=VERTEX_POINT('',#35092);
#5273=VERTEX_POINT('',#35096);
#5274=VERTEX_POINT('',#35098);
#5275=VERTEX_POINT('',#35102);
#5276=VERTEX_POINT('',#35104);
#5277=VERTEX_POINT('',#35108);
#5278=VERTEX_POINT('',#35110);
#5279=VERTEX_POINT('',#35114);
#5280=VERTEX_POINT('',#35116);
#5281=VERTEX_POINT('',#35120);
#5282=VERTEX_POINT('',#35122);
#5283=VERTEX_POINT('',#35132);
#5284=VERTEX_POINT('',#35134);
#5285=VERTEX_POINT('',#35138);
#5286=VERTEX_POINT('',#35140);
#5287=VERTEX_POINT('',#35144);
#5288=VERTEX_POINT('',#35146);
#5289=VERTEX_POINT('',#35150);
#5290=VERTEX_POINT('',#35152);
#5291=VERTEX_POINT('',#35156);
#5292=VERTEX_POINT('',#35158);
#5293=VERTEX_POINT('',#35162);
#5294=VERTEX_POINT('',#35164);
#5295=VERTEX_POINT('',#35168);
#5296=VERTEX_POINT('',#35170);
#5297=VERTEX_POINT('',#35174);
#5298=VERTEX_POINT('',#35176);
#5299=VERTEX_POINT('',#35178);
#5300=VERTEX_POINT('',#35180);
#5301=VERTEX_POINT('',#35182);
#5302=VERTEX_POINT('',#35184);
#5303=VERTEX_POINT('',#35186);
#5304=VERTEX_POINT('',#35188);
#5305=VERTEX_POINT('',#35190);
#5306=VERTEX_POINT('',#35192);
#5307=VERTEX_POINT('',#35194);
#5308=VERTEX_POINT('',#35196);
#5309=VERTEX_POINT('',#35198);
#5310=VERTEX_POINT('',#35200);
#5311=VERTEX_POINT('',#35202);
#5312=VERTEX_POINT('',#35204);
#5313=VERTEX_POINT('',#35206);
#5314=VERTEX_POINT('',#35208);
#5315=VERTEX_POINT('',#35210);
#5316=VERTEX_POINT('',#35212);
#5317=VERTEX_POINT('',#35214);
#5318=VERTEX_POINT('',#35216);
#5319=VERTEX_POINT('',#35218);
#5320=VERTEX_POINT('',#35220);
#5321=VERTEX_POINT('',#35222);
#5322=VERTEX_POINT('',#35224);
#5323=VERTEX_POINT('',#35226);
#5324=VERTEX_POINT('',#35228);
#5325=VERTEX_POINT('',#35230);
#5326=VERTEX_POINT('',#35232);
#5327=VERTEX_POINT('',#35234);
#5328=VERTEX_POINT('',#35236);
#5329=VERTEX_POINT('',#35238);
#5330=VERTEX_POINT('',#35240);
#5331=VERTEX_POINT('',#35242);
#5332=VERTEX_POINT('',#35244);
#5333=VERTEX_POINT('',#35246);
#5334=VERTEX_POINT('',#35248);
#5335=VERTEX_POINT('',#35250);
#5336=VERTEX_POINT('',#35252);
#5337=VERTEX_POINT('',#35255);
#5338=VERTEX_POINT('',#35257);
#5339=VERTEX_POINT('',#35259);
#5340=VERTEX_POINT('',#35261);
#5341=VERTEX_POINT('',#35264);
#5342=VERTEX_POINT('',#35267);
#5343=VERTEX_POINT('',#35271);
#5344=VERTEX_POINT('',#35275);
#5345=VERTEX_POINT('',#35277);
#5346=VERTEX_POINT('',#35281);
#5347=VERTEX_POINT('',#35283);
#5348=VERTEX_POINT('',#35287);
#5349=VERTEX_POINT('',#35289);
#5350=VERTEX_POINT('',#35293);
#5351=VERTEX_POINT('',#35297);
#5352=VERTEX_POINT('',#35299);
#5353=VERTEX_POINT('',#35303);
#5354=VERTEX_POINT('',#35305);
#5355=VERTEX_POINT('',#35311);
#5356=VERTEX_POINT('',#35315);
#5357=VERTEX_POINT('',#35319);
#5358=VERTEX_POINT('',#35323);
#5359=VERTEX_POINT('',#35327);
#5360=VERTEX_POINT('',#35331);
#5361=VERTEX_POINT('',#35335);
#5362=VERTEX_POINT('',#35339);
#5363=VERTEX_POINT('',#35343);
#5364=VERTEX_POINT('',#35347);
#5365=VERTEX_POINT('',#35353);
#5366=VERTEX_POINT('',#35355);
#5367=VERTEX_POINT('',#35363);
#5368=VERTEX_POINT('',#35367);
#5369=VERTEX_POINT('',#35371);
#5370=VERTEX_POINT('',#35377);
#5371=VERTEX_POINT('',#35379);
#5372=VERTEX_POINT('',#35385);
#5373=VERTEX_POINT('',#35389);
#5374=VERTEX_POINT('',#35393);
#5375=VERTEX_POINT('',#35397);
#5376=VERTEX_POINT('',#35401);
#5377=VERTEX_POINT('',#35405);
#5378=VERTEX_POINT('',#35409);
#5379=VERTEX_POINT('',#35413);
#5380=VERTEX_POINT('',#35417);
#5381=VERTEX_POINT('',#35421);
#5382=VERTEX_POINT('',#35429);
#5383=VERTEX_POINT('',#35433);
#5384=VERTEX_POINT('',#35437);
#5385=VERTEX_POINT('',#35441);
#5386=VERTEX_POINT('',#35445);
#6556=EDGE_CURVE('',#5199,#5200,#2812,.T.);
#6557=EDGE_CURVE('',#5200,#5201,#2813,.T.);
#6558=EDGE_CURVE('',#5201,#5202,#2814,.T.);
#6559=EDGE_CURVE('',#5199,#5202,#2815,.T.);
#6560=EDGE_CURVE('',#5203,#5204,#2816,.T.);
#6561=EDGE_CURVE('',#5204,#5205,#2817,.T.);
#6562=EDGE_CURVE('',#5205,#5206,#2818,.T.);
#6563=EDGE_CURVE('',#5203,#5206,#2819,.T.);
#6564=EDGE_CURVE('',#5207,#5208,#2820,.T.);
#6565=EDGE_CURVE('',#5209,#5207,#2821,.T.);
#6566=EDGE_CURVE('',#5209,#5210,#2822,.T.);
#6567=EDGE_CURVE('',#5210,#5208,#2823,.F.);
#6568=EDGE_CURVE('',#5211,#5212,#2824,.T.);
#6569=EDGE_CURVE('',#5212,#5213,#2825,.F.);
#6570=EDGE_CURVE('',#5214,#5213,#2826,.T.);
#6571=EDGE_CURVE('',#5211,#5214,#2827,.T.);
#6572=EDGE_CURVE('',#5215,#5216,#2828,.T.);
#6573=EDGE_CURVE('',#5217,#5215,#2829,.T.);
#6574=EDGE_CURVE('',#5217,#5218,#2830,.T.);
#6575=EDGE_CURVE('',#5218,#5216,#2831,.F.);
#6576=EDGE_CURVE('',#5219,#5219,#4441,.F.);
#6577=EDGE_CURVE('',#5219,#5220,#2832,.T.);
#6578=EDGE_CURVE('',#5220,#5220,#4442,.T.);
#6579=EDGE_CURVE('',#5221,#5222,#2833,.T.);
#6580=EDGE_CURVE('',#5222,#5223,#2834,.F.);
#6581=EDGE_CURVE('',#5224,#5223,#2835,.T.);
#6582=EDGE_CURVE('',#5221,#5224,#2836,.T.);
#6583=EDGE_CURVE('',#5225,#5226,#2837,.T.);
#6584=EDGE_CURVE('',#5226,#5227,#2838,.T.);
#6585=EDGE_CURVE('',#5227,#5228,#2839,.F.);
#6586=EDGE_CURVE('',#5225,#5228,#2840,.T.);
#6587=EDGE_CURVE('',#5226,#5224,#2841,.T.);
#6588=EDGE_CURVE('',#5223,#5227,#2842,.F.);
#6589=EDGE_CURVE('',#5229,#5217,#2843,.T.);
#6590=EDGE_CURVE('',#5229,#5230,#2844,.T.);
#6591=EDGE_CURVE('',#5230,#5218,#2845,.F.);
#6592=EDGE_CURVE('',#5231,#5229,#2846,.T.);
#6593=EDGE_CURVE('',#5231,#5232,#2847,.T.);
#6594=EDGE_CURVE('',#5232,#5230,#2848,.F.);
#6595=EDGE_CURVE('',#5231,#5233,#2849,.T.);
#6596=EDGE_CURVE('',#5233,#5234,#2850,.T.);
#6597=EDGE_CURVE('',#5234,#5232,#2851,.F.);
#6598=EDGE_CURVE('',#5233,#5235,#2852,.T.);
#6599=EDGE_CURVE('',#5235,#5236,#2853,.T.);
#6600=EDGE_CURVE('',#5236,#5234,#2854,.F.);
#6601=EDGE_CURVE('',#5237,#5235,#2855,.T.);
#6602=EDGE_CURVE('',#5237,#5238,#2856,.T.);
#6603=EDGE_CURVE('',#5238,#5236,#2857,.F.);
#6604=EDGE_CURVE('',#5239,#5237,#2858,.T.);
#6605=EDGE_CURVE('',#5239,#5240,#2859,.T.);
#6606=EDGE_CURVE('',#5240,#5238,#2860,.F.);
#6607=EDGE_CURVE('',#5241,#5239,#4443,.T.);
#6608=EDGE_CURVE('',#5241,#5242,#2861,.T.);
#6609=EDGE_CURVE('',#5242,#5240,#4444,.F.);
#6610=EDGE_CURVE('',#5243,#5241,#2862,.T.);
#6611=EDGE_CURVE('',#5243,#5244,#2863,.T.);
#6612=EDGE_CURVE('',#5244,#5242,#2864,.F.);
#6613=EDGE_CURVE('',#5243,#5245,#2865,.T.);
#6614=EDGE_CURVE('',#5245,#5246,#2866,.T.);
#6615=EDGE_CURVE('',#5246,#5244,#2867,.F.);
#6616=EDGE_CURVE('',#5247,#5245,#2868,.T.);
#6617=EDGE_CURVE('',#5247,#5248,#2869,.T.);
#6618=EDGE_CURVE('',#5248,#5246,#2870,.F.);
#6619=EDGE_CURVE('',#5225,#5247,#2871,.T.);
#6620=EDGE_CURVE('',#5228,#5248,#2872,.F.);
#6621=EDGE_CURVE('',#5249,#5250,#2873,.T.);
#6622=EDGE_CURVE('',#5250,#5251,#2874,.T.);
#6623=EDGE_CURVE('',#5251,#5252,#2875,.F.);
#6624=EDGE_CURVE('',#5249,#5252,#2876,.T.);
#6625=EDGE_CURVE('',#5250,#5214,#2877,.T.);
#6626=EDGE_CURVE('',#5213,#5251,#2878,.F.);
#6627=EDGE_CURVE('',#5203,#5209,#2879,.T.);
#6628=EDGE_CURVE('',#5206,#5210,#2880,.F.);
#6629=EDGE_CURVE('',#5253,#5254,#2881,.T.);
#6630=EDGE_CURVE('',#5254,#5255,#2882,.T.);
#6631=EDGE_CURVE('',#5255,#5256,#2883,.F.);
#6632=EDGE_CURVE('',#5253,#5256,#2884,.T.);
#6633=EDGE_CURVE('',#5257,#5254,#2885,.T.);
#6634=EDGE_CURVE('',#5257,#5258,#2886,.T.);
#6635=EDGE_CURVE('',#5258,#5255,#2887,.F.);
#6636=EDGE_CURVE('',#5249,#5257,#2888,.T.);
#6637=EDGE_CURVE('',#5252,#5258,#2889,.F.);
#6638=EDGE_CURVE('',#5259,#5260,#2890,.T.);
#6639=EDGE_CURVE('',#5260,#5261,#2891,.T.);
#6640=EDGE_CURVE('',#5261,#5262,#2892,.F.);
#6641=EDGE_CURVE('',#5259,#5262,#2893,.T.);
#6642=EDGE_CURVE('',#5260,#5215,#2894,.T.);
#6643=EDGE_CURVE('',#5216,#5261,#2895,.F.);
#6644=EDGE_CURVE('',#5263,#5211,#2896,.T.);
#6645=EDGE_CURVE('',#5263,#5264,#2897,.T.);
#6646=EDGE_CURVE('',#5264,#5212,#2898,.F.);
#6647=EDGE_CURVE('',#5265,#5263,#2899,.T.);
#6648=EDGE_CURVE('',#5265,#5266,#2900,.T.);
#6649=EDGE_CURVE('',#5266,#5264,#2901,.F.);
#6650=EDGE_CURVE('',#5265,#5267,#2902,.T.);
#6651=EDGE_CURVE('',#5267,#5268,#2903,.T.);
#6652=EDGE_CURVE('',#5268,#5266,#2904,.F.);
#6653=EDGE_CURVE('',#5267,#5269,#2905,.T.);
#6654=EDGE_CURVE('',#5269,#5270,#2906,.T.);
#6655=EDGE_CURVE('',#5270,#5268,#2907,.F.);
#6656=EDGE_CURVE('',#5271,#5269,#2908,.T.);
#6657=EDGE_CURVE('',#5271,#5272,#2909,.T.);
#6658=EDGE_CURVE('',#5272,#5270,#2910,.F.);
#6659=EDGE_CURVE('',#5273,#5271,#2911,.T.);
#6660=EDGE_CURVE('',#5273,#5274,#2912,.T.);
#6661=EDGE_CURVE('',#5274,#5272,#2913,.F.);
#6662=EDGE_CURVE('',#5275,#5273,#4445,.T.);
#6663=EDGE_CURVE('',#5275,#5276,#2914,.T.);
#6664=EDGE_CURVE('',#5276,#5274,#4446,.F.);
#6665=EDGE_CURVE('',#5277,#5275,#2915,.T.);
#6666=EDGE_CURVE('',#5277,#5278,#2916,.T.);
#6667=EDGE_CURVE('',#5278,#5276,#2917,.F.);
#6668=EDGE_CURVE('',#5277,#5279,#2918,.T.);
#6669=EDGE_CURVE('',#5279,#5280,#2919,.T.);
#6670=EDGE_CURVE('',#5280,#5278,#2920,.F.);
#6671=EDGE_CURVE('',#5281,#5279,#2921,.T.);
#6672=EDGE_CURVE('',#5281,#5282,#2922,.T.);
#6673=EDGE_CURVE('',#5282,#5280,#2923,.F.);
#6674=EDGE_CURVE('',#5259,#5281,#2924,.T.);
#6675=EDGE_CURVE('',#5262,#5282,#2925,.F.);
#6676=EDGE_CURVE('',#5200,#5207,#2926,.T.);
#6677=EDGE_CURVE('',#5208,#5201,#2927,.F.);
#6678=EDGE_CURVE('',#5283,#5221,#2928,.T.);
#6679=EDGE_CURVE('',#5283,#5284,#2929,.T.);
#6680=EDGE_CURVE('',#5284,#5222,#2930,.F.);
#6681=EDGE_CURVE('',#5285,#5283,#2931,.T.);
#6682=EDGE_CURVE('',#5285,#5286,#2932,.T.);
#6683=EDGE_CURVE('',#5286,#5284,#2933,.F.);
#6684=EDGE_CURVE('',#5285,#5287,#2934,.T.);
#6685=EDGE_CURVE('',#5287,#5288,#2935,.T.);
#6686=EDGE_CURVE('',#5288,#5286,#2936,.F.);
#6687=EDGE_CURVE('',#5287,#5289,#2937,.T.);
#6688=EDGE_CURVE('',#5289,#5290,#2938,.T.);
#6689=EDGE_CURVE('',#5290,#5288,#2939,.F.);
#6690=EDGE_CURVE('',#5291,#5289,#2940,.T.);
#6691=EDGE_CURVE('',#5291,#5292,#2941,.T.);
#6692=EDGE_CURVE('',#5292,#5290,#2942,.F.);
#6693=EDGE_CURVE('',#5199,#5293,#2943,.T.);
#6694=EDGE_CURVE('',#5202,#5294,#2944,.T.);
#6695=EDGE_CURVE('',#5293,#5294,#2945,.T.);
#6696=EDGE_CURVE('',#5293,#5295,#2946,.T.);
#6697=EDGE_CURVE('',#5296,#5294,#2947,.F.);
#6698=EDGE_CURVE('',#5295,#5296,#2948,.T.);
#6699=EDGE_CURVE('',#5297,#5291,#2949,.T.);
#6700=EDGE_CURVE('',#5298,#5253,#2950,.T.);
#6701=EDGE_CURVE('',#5298,#5299,#2951,.T.);
#6702=EDGE_CURVE('',#5300,#5299,#2952,.T.);
#6703=EDGE_CURVE('',#5301,#5300,#2953,.T.);
#6704=EDGE_CURVE('',#5301,#5302,#2954,.T.);
#6705=EDGE_CURVE('',#5302,#5303,#2955,.T.);
#6706=EDGE_CURVE('',#5304,#5303,#2956,.T.);
#6707=EDGE_CURVE('',#5305,#5304,#2957,.T.);
#6708=EDGE_CURVE('',#5306,#5305,#2958,.T.);
#6709=EDGE_CURVE('',#5306,#5307,#2959,.T.);
#6710=EDGE_CURVE('',#5307,#5308,#2960,.T.);
#6711=EDGE_CURVE('',#5309,#5308,#2961,.T.);
#6712=EDGE_CURVE('',#5310,#5309,#2962,.T.);
#6713=EDGE_CURVE('',#5311,#5310,#4447,.T.);
#6714=EDGE_CURVE('',#5312,#5311,#2963,.T.);
#6715=EDGE_CURVE('',#5312,#5313,#2964,.T.);
#6716=EDGE_CURVE('',#5314,#5313,#2965,.T.);
#6717=EDGE_CURVE('',#5315,#5314,#2966,.T.);
#6718=EDGE_CURVE('',#5315,#5316,#2967,.T.);
#6719=EDGE_CURVE('',#5316,#5317,#2968,.T.);
#6720=EDGE_CURVE('',#5318,#5317,#2969,.T.);
#6721=EDGE_CURVE('',#5319,#5318,#2970,.T.);
#6722=EDGE_CURVE('',#5320,#5319,#2971,.T.);
#6723=EDGE_CURVE('',#5320,#5321,#2972,.T.);
#6724=EDGE_CURVE('',#5321,#5322,#2973,.T.);
#6725=EDGE_CURVE('',#5323,#5322,#2974,.T.);
#6726=EDGE_CURVE('',#5324,#5323,#2975,.T.);
#6727=EDGE_CURVE('',#5325,#5324,#4448,.T.);
#6728=EDGE_CURVE('',#5326,#5325,#2976,.T.);
#6729=EDGE_CURVE('',#5326,#5327,#2977,.T.);
#6730=EDGE_CURVE('',#5328,#5327,#2978,.T.);
#6731=EDGE_CURVE('',#5329,#5328,#2979,.T.);
#6732=EDGE_CURVE('',#5329,#5330,#2980,.T.);
#6733=EDGE_CURVE('',#5330,#5331,#2981,.T.);
#6734=EDGE_CURVE('',#5332,#5331,#2982,.T.);
#6735=EDGE_CURVE('',#5333,#5332,#2983,.T.);
#6736=EDGE_CURVE('',#5334,#5333,#2984,.T.);
#6737=EDGE_CURVE('',#5334,#5335,#2985,.T.);
#6738=EDGE_CURVE('',#5335,#5336,#2986,.T.);
#6739=EDGE_CURVE('',#5297,#5336,#2987,.T.);
#6740=EDGE_CURVE('',#5295,#5337,#2988,.T.);
#6741=EDGE_CURVE('',#5338,#5337,#2989,.T.);
#6742=EDGE_CURVE('',#5339,#5338,#2990,.T.);
#6743=EDGE_CURVE('',#5339,#5340,#2991,.T.);
#6744=EDGE_CURVE('',#5340,#5204,#2992,.T.);
#6745=EDGE_CURVE('',#5341,#5341,#4449,.T.);
#6746=EDGE_CURVE('',#5340,#5342,#2993,.T.);
#6747=EDGE_CURVE('',#5342,#5205,#2994,.T.);
#6748=EDGE_CURVE('',#5339,#5343,#2995,.T.);
#6749=EDGE_CURVE('',#5342,#5343,#2996,.F.);
#6750=EDGE_CURVE('',#5337,#5344,#2997,.T.);
#6751=EDGE_CURVE('',#5345,#5344,#2998,.T.);
#6752=EDGE_CURVE('',#5338,#5345,#2999,.T.);
#6753=EDGE_CURVE('',#5304,#5346,#3000,.T.);
#6754=EDGE_CURVE('',#5303,#5347,#3001,.T.);
#6755=EDGE_CURVE('',#5346,#5347,#3002,.T.);
#6756=EDGE_CURVE('',#5317,#5348,#3003,.T.);
#6757=EDGE_CURVE('',#5349,#5348,#3004,.T.);
#6758=EDGE_CURVE('',#5318,#5349,#3005,.T.);
#6759=EDGE_CURVE('',#5341,#5350,#3006,.T.);
#6760=EDGE_CURVE('',#5350,#5350,#4450,.T.);
#6761=EDGE_CURVE('',#5332,#5351,#3007,.T.);
#6762=EDGE_CURVE('',#5331,#5352,#3008,.T.);
#6763=EDGE_CURVE('',#5351,#5352,#3009,.T.);
#6764=EDGE_CURVE('',#5329,#5353,#3010,.T.);
#6765=EDGE_CURVE('',#5354,#5353,#3011,.T.);
#6766=EDGE_CURVE('',#5330,#5354,#3012,.T.);
#6767=EDGE_CURVE('',#5352,#5354,#3013,.T.);
#6768=EDGE_CURVE('',#5355,#5349,#3014,.T.);
#6769=EDGE_CURVE('',#5319,#5355,#3015,.T.);
#6770=EDGE_CURVE('',#5356,#5355,#3016,.T.);
#6771=EDGE_CURVE('',#5320,#5356,#3017,.T.);
#6772=EDGE_CURVE('',#5357,#5356,#3018,.T.);
#6773=EDGE_CURVE('',#5321,#5357,#3019,.T.);
#6774=EDGE_CURVE('',#5358,#5357,#3020,.T.);
#6775=EDGE_CURVE('',#5322,#5358,#3021,.T.);
#6776=EDGE_CURVE('',#5359,#5358,#3022,.T.);
#6777=EDGE_CURVE('',#5323,#5359,#3023,.T.);
#6778=EDGE_CURVE('',#5360,#5359,#3024,.T.);
#6779=EDGE_CURVE('',#5324,#5360,#3025,.T.);
#6780=EDGE_CURVE('',#5361,#5360,#4451,.T.);
#6781=EDGE_CURVE('',#5325,#5361,#3026,.T.);
#6782=EDGE_CURVE('',#5362,#5361,#3027,.T.);
#6783=EDGE_CURVE('',#5326,#5362,#3028,.T.);
#6784=EDGE_CURVE('',#5363,#5362,#3029,.T.);
#6785=EDGE_CURVE('',#5327,#5363,#3030,.T.);
#6786=EDGE_CURVE('',#5364,#5363,#3031,.T.);
#6787=EDGE_CURVE('',#5328,#5364,#3032,.T.);
#6788=EDGE_CURVE('',#5353,#5364,#3033,.T.);
#6789=EDGE_CURVE('',#5301,#5365,#3034,.T.);
#6790=EDGE_CURVE('',#5366,#5365,#3035,.T.);
#6791=EDGE_CURVE('',#5302,#5366,#3036,.T.);
#6792=EDGE_CURVE('',#5347,#5366,#3037,.T.);
#6793=EDGE_CURVE('',#5343,#5345,#3038,.T.);
#6794=EDGE_CURVE('',#5367,#5256,#3039,.T.);
#6795=EDGE_CURVE('',#5298,#5367,#3040,.T.);
#6796=EDGE_CURVE('',#5368,#5367,#3041,.T.);
#6797=EDGE_CURVE('',#5299,#5368,#3042,.T.);
#6798=EDGE_CURVE('',#5369,#5368,#3043,.T.);
#6799=EDGE_CURVE('',#5300,#5369,#3044,.T.);
#6800=EDGE_CURVE('',#5365,#5369,#3045,.T.);
#6801=EDGE_CURVE('',#5315,#5370,#3046,.T.);
#6802=EDGE_CURVE('',#5371,#5370,#3047,.T.);
#6803=EDGE_CURVE('',#5316,#5371,#3048,.T.);
#6804=EDGE_CURVE('',#5348,#5371,#3049,.T.);
#6805=EDGE_CURVE('',#5372,#5346,#3050,.T.);
#6806=EDGE_CURVE('',#5305,#5372,#3051,.T.);
#6807=EDGE_CURVE('',#5373,#5372,#3052,.T.);
#6808=EDGE_CURVE('',#5306,#5373,#3053,.T.);
#6809=EDGE_CURVE('',#5374,#5373,#3054,.T.);
#6810=EDGE_CURVE('',#5307,#5374,#3055,.T.);
#6811=EDGE_CURVE('',#5375,#5374,#3056,.T.);
#6812=EDGE_CURVE('',#5308,#5375,#3057,.T.);
#6813=EDGE_CURVE('',#5376,#5375,#3058,.T.);
#6814=EDGE_CURVE('',#5309,#5376,#3059,.T.);
#6815=EDGE_CURVE('',#5377,#5376,#3060,.T.);
#6816=EDGE_CURVE('',#5310,#5377,#3061,.T.);
#6817=EDGE_CURVE('',#5378,#5377,#4452,.T.);
#6818=EDGE_CURVE('',#5311,#5378,#3062,.T.);
#6819=EDGE_CURVE('',#5379,#5378,#3063,.T.);
#6820=EDGE_CURVE('',#5312,#5379,#3064,.T.);
#6821=EDGE_CURVE('',#5380,#5379,#3065,.T.);
#6822=EDGE_CURVE('',#5313,#5380,#3066,.T.);
#6823=EDGE_CURVE('',#5381,#5380,#3067,.T.);
#6824=EDGE_CURVE('',#5314,#5381,#3068,.T.);
#6825=EDGE_CURVE('',#5370,#5381,#3069,.T.);
#6826=EDGE_CURVE('',#5344,#5296,#3070,.T.);
#6827=EDGE_CURVE('',#5382,#5351,#3071,.T.);
#6828=EDGE_CURVE('',#5333,#5382,#3072,.T.);
#6829=EDGE_CURVE('',#5383,#5382,#3073,.T.);
#6830=EDGE_CURVE('',#5334,#5383,#3074,.T.);
#6831=EDGE_CURVE('',#5384,#5383,#3075,.T.);
#6832=EDGE_CURVE('',#5335,#5384,#3076,.T.);
#6833=EDGE_CURVE('',#5385,#5384,#3077,.T.);
#6834=EDGE_CURVE('',#5336,#5385,#3078,.T.);
#6835=EDGE_CURVE('',#5386,#5385,#3079,.T.);
#6836=EDGE_CURVE('',#5297,#5386,#3080,.T.);
#6837=EDGE_CURVE('',#5386,#5292,#3081,.F.);
#9050=ORIENTED_EDGE('',*,*,#6556,.T.);
#9051=ORIENTED_EDGE('',*,*,#6557,.T.);
#9052=ORIENTED_EDGE('',*,*,#6558,.T.);
#9053=ORIENTED_EDGE('',*,*,#6559,.F.);
#9054=ORIENTED_EDGE('',*,*,#6560,.T.);
#9055=ORIENTED_EDGE('',*,*,#6561,.T.);
#9056=ORIENTED_EDGE('',*,*,#6562,.T.);
#9057=ORIENTED_EDGE('',*,*,#6563,.F.);
#9058=ORIENTED_EDGE('',*,*,#6564,.F.);
#9059=ORIENTED_EDGE('',*,*,#6565,.F.);
#9060=ORIENTED_EDGE('',*,*,#6566,.T.);
#9061=ORIENTED_EDGE('',*,*,#6567,.T.);
#9062=ORIENTED_EDGE('',*,*,#6568,.T.);
#9063=ORIENTED_EDGE('',*,*,#6569,.T.);
#9064=ORIENTED_EDGE('',*,*,#6570,.F.);
#9065=ORIENTED_EDGE('',*,*,#6571,.F.);
#9066=ORIENTED_EDGE('',*,*,#6572,.F.);
#9067=ORIENTED_EDGE('',*,*,#6573,.F.);
#9068=ORIENTED_EDGE('',*,*,#6574,.T.);
#9069=ORIENTED_EDGE('',*,*,#6575,.T.);
#9070=ORIENTED_EDGE('',*,*,#6576,.T.);
#9071=ORIENTED_EDGE('',*,*,#6577,.T.);
#9072=ORIENTED_EDGE('',*,*,#6578,.F.);
#9073=ORIENTED_EDGE('',*,*,#6577,.F.);
#9074=ORIENTED_EDGE('',*,*,#6579,.T.);
#9075=ORIENTED_EDGE('',*,*,#6580,.T.);
#9076=ORIENTED_EDGE('',*,*,#6581,.F.);
#9077=ORIENTED_EDGE('',*,*,#6582,.F.);
#9078=ORIENTED_EDGE('',*,*,#6583,.T.);
#9079=ORIENTED_EDGE('',*,*,#6584,.T.);
#9080=ORIENTED_EDGE('',*,*,#6585,.T.);
#9081=ORIENTED_EDGE('',*,*,#6586,.F.);
#9082=ORIENTED_EDGE('',*,*,#6587,.T.);
#9083=ORIENTED_EDGE('',*,*,#6581,.T.);
#9084=ORIENTED_EDGE('',*,*,#6588,.T.);
#9085=ORIENTED_EDGE('',*,*,#6584,.F.);
#9086=ORIENTED_EDGE('',*,*,#6589,.F.);
#9087=ORIENTED_EDGE('',*,*,#6590,.T.);
#9088=ORIENTED_EDGE('',*,*,#6591,.T.);
#9089=ORIENTED_EDGE('',*,*,#6574,.F.);
#9090=ORIENTED_EDGE('',*,*,#6592,.F.);
#9091=ORIENTED_EDGE('',*,*,#6593,.T.);
#9092=ORIENTED_EDGE('',*,*,#6594,.T.);
#9093=ORIENTED_EDGE('',*,*,#6590,.F.);
#9094=ORIENTED_EDGE('',*,*,#6595,.T.);
#9095=ORIENTED_EDGE('',*,*,#6596,.T.);
#9096=ORIENTED_EDGE('',*,*,#6597,.T.);
#9097=ORIENTED_EDGE('',*,*,#6593,.F.);
#9098=ORIENTED_EDGE('',*,*,#6598,.T.);
#9099=ORIENTED_EDGE('',*,*,#6599,.T.);
#9100=ORIENTED_EDGE('',*,*,#6600,.T.);
#9101=ORIENTED_EDGE('',*,*,#6596,.F.);
#9102=ORIENTED_EDGE('',*,*,#6601,.F.);
#9103=ORIENTED_EDGE('',*,*,#6602,.T.);
#9104=ORIENTED_EDGE('',*,*,#6603,.T.);
#9105=ORIENTED_EDGE('',*,*,#6599,.F.);
#9106=ORIENTED_EDGE('',*,*,#6604,.F.);
#9107=ORIENTED_EDGE('',*,*,#6605,.T.);
#9108=ORIENTED_EDGE('',*,*,#6606,.T.);
#9109=ORIENTED_EDGE('',*,*,#6602,.F.);
#9110=ORIENTED_EDGE('',*,*,#6607,.F.);
#9111=ORIENTED_EDGE('',*,*,#6608,.T.);
#9112=ORIENTED_EDGE('',*,*,#6609,.T.);
#9113=ORIENTED_EDGE('',*,*,#6605,.F.);
#9114=ORIENTED_EDGE('',*,*,#6610,.F.);
#9115=ORIENTED_EDGE('',*,*,#6611,.T.);
#9116=ORIENTED_EDGE('',*,*,#6612,.T.);
#9117=ORIENTED_EDGE('',*,*,#6608,.F.);
#9118=ORIENTED_EDGE('',*,*,#6613,.T.);
#9119=ORIENTED_EDGE('',*,*,#6614,.T.);
#9120=ORIENTED_EDGE('',*,*,#6615,.T.);
#9121=ORIENTED_EDGE('',*,*,#6611,.F.);
#9122=ORIENTED_EDGE('',*,*,#6616,.F.);
#9123=ORIENTED_EDGE('',*,*,#6617,.T.);
#9124=ORIENTED_EDGE('',*,*,#6618,.T.);
#9125=ORIENTED_EDGE('',*,*,#6614,.F.);
#9126=ORIENTED_EDGE('',*,*,#6619,.F.);
#9127=ORIENTED_EDGE('',*,*,#6586,.T.);
#9128=ORIENTED_EDGE('',*,*,#6620,.T.);
#9129=ORIENTED_EDGE('',*,*,#6617,.F.);
#9130=ORIENTED_EDGE('',*,*,#6621,.T.);
#9131=ORIENTED_EDGE('',*,*,#6622,.T.);
#9132=ORIENTED_EDGE('',*,*,#6623,.T.);
#9133=ORIENTED_EDGE('',*,*,#6624,.F.);
#9134=ORIENTED_EDGE('',*,*,#6625,.T.);
#9135=ORIENTED_EDGE('',*,*,#6570,.T.);
#9136=ORIENTED_EDGE('',*,*,#6626,.T.);
#9137=ORIENTED_EDGE('',*,*,#6622,.F.);
#9138=ORIENTED_EDGE('',*,*,#6627,.F.);
#9139=ORIENTED_EDGE('',*,*,#6563,.T.);
#9140=ORIENTED_EDGE('',*,*,#6628,.T.);
#9141=ORIENTED_EDGE('',*,*,#6566,.F.);
#9142=ORIENTED_EDGE('',*,*,#6629,.T.);
#9143=ORIENTED_EDGE('',*,*,#6630,.T.);
#9144=ORIENTED_EDGE('',*,*,#6631,.T.);
#9145=ORIENTED_EDGE('',*,*,#6632,.F.);
#9146=ORIENTED_EDGE('',*,*,#6633,.F.);
#9147=ORIENTED_EDGE('',*,*,#6634,.T.);
#9148=ORIENTED_EDGE('',*,*,#6635,.T.);
#9149=ORIENTED_EDGE('',*,*,#6630,.F.);
#9150=ORIENTED_EDGE('',*,*,#6636,.F.);
#9151=ORIENTED_EDGE('',*,*,#6624,.T.);
#9152=ORIENTED_EDGE('',*,*,#6637,.T.);
#9153=ORIENTED_EDGE('',*,*,#6634,.F.);
#9154=ORIENTED_EDGE('',*,*,#6638,.T.);
#9155=ORIENTED_EDGE('',*,*,#6639,.T.);
#9156=ORIENTED_EDGE('',*,*,#6640,.T.);
#9157=ORIENTED_EDGE('',*,*,#6641,.F.);
#9158=ORIENTED_EDGE('',*,*,#6642,.T.);
#9159=ORIENTED_EDGE('',*,*,#6572,.T.);
#9160=ORIENTED_EDGE('',*,*,#6643,.T.);
#9161=ORIENTED_EDGE('',*,*,#6639,.F.);
#9162=ORIENTED_EDGE('',*,*,#6644,.F.);
#9163=ORIENTED_EDGE('',*,*,#6645,.T.);
#9164=ORIENTED_EDGE('',*,*,#6646,.T.);
#9165=ORIENTED_EDGE('',*,*,#6568,.F.);
#9166=ORIENTED_EDGE('',*,*,#6647,.F.);
#9167=ORIENTED_EDGE('',*,*,#6648,.T.);
#9168=ORIENTED_EDGE('',*,*,#6649,.T.);
#9169=ORIENTED_EDGE('',*,*,#6645,.F.);
#9170=ORIENTED_EDGE('',*,*,#6650,.T.);
#9171=ORIENTED_EDGE('',*,*,#6651,.T.);
#9172=ORIENTED_EDGE('',*,*,#6652,.T.);
#9173=ORIENTED_EDGE('',*,*,#6648,.F.);
#9174=ORIENTED_EDGE('',*,*,#6653,.T.);
#9175=ORIENTED_EDGE('',*,*,#6654,.T.);
#9176=ORIENTED_EDGE('',*,*,#6655,.T.);
#9177=ORIENTED_EDGE('',*,*,#6651,.F.);
#9178=ORIENTED_EDGE('',*,*,#6656,.F.);
#9179=ORIENTED_EDGE('',*,*,#6657,.T.);
#9180=ORIENTED_EDGE('',*,*,#6658,.T.);
#9181=ORIENTED_EDGE('',*,*,#6654,.F.);
#9182=ORIENTED_EDGE('',*,*,#6659,.F.);
#9183=ORIENTED_EDGE('',*,*,#6660,.T.);
#9184=ORIENTED_EDGE('',*,*,#6661,.T.);
#9185=ORIENTED_EDGE('',*,*,#6657,.F.);
#9186=ORIENTED_EDGE('',*,*,#6662,.F.);
#9187=ORIENTED_EDGE('',*,*,#6663,.T.);
#9188=ORIENTED_EDGE('',*,*,#6664,.T.);
#9189=ORIENTED_EDGE('',*,*,#6660,.F.);
#9190=ORIENTED_EDGE('',*,*,#6665,.F.);
#9191=ORIENTED_EDGE('',*,*,#6666,.T.);
#9192=ORIENTED_EDGE('',*,*,#6667,.T.);
#9193=ORIENTED_EDGE('',*,*,#6663,.F.);
#9194=ORIENTED_EDGE('',*,*,#6668,.T.);
#9195=ORIENTED_EDGE('',*,*,#6669,.T.);
#9196=ORIENTED_EDGE('',*,*,#6670,.T.);
#9197=ORIENTED_EDGE('',*,*,#6666,.F.);
#9198=ORIENTED_EDGE('',*,*,#6671,.F.);
#9199=ORIENTED_EDGE('',*,*,#6672,.T.);
#9200=ORIENTED_EDGE('',*,*,#6673,.T.);
#9201=ORIENTED_EDGE('',*,*,#6669,.F.);
#9202=ORIENTED_EDGE('',*,*,#6674,.F.);
#9203=ORIENTED_EDGE('',*,*,#6641,.T.);
#9204=ORIENTED_EDGE('',*,*,#6675,.T.);
#9205=ORIENTED_EDGE('',*,*,#6672,.F.);
#9206=ORIENTED_EDGE('',*,*,#6676,.T.);
#9207=ORIENTED_EDGE('',*,*,#6564,.T.);
#9208=ORIENTED_EDGE('',*,*,#6677,.T.);
#9209=ORIENTED_EDGE('',*,*,#6557,.F.);
#9210=ORIENTED_EDGE('',*,*,#6678,.F.);
#9211=ORIENTED_EDGE('',*,*,#6679,.T.);
#9212=ORIENTED_EDGE('',*,*,#6680,.T.);
#9213=ORIENTED_EDGE('',*,*,#6579,.F.);
#9214=ORIENTED_EDGE('',*,*,#6681,.F.);
#9215=ORIENTED_EDGE('',*,*,#6682,.T.);
#9216=ORIENTED_EDGE('',*,*,#6683,.T.);
#9217=ORIENTED_EDGE('',*,*,#6679,.F.);
#9218=ORIENTED_EDGE('',*,*,#6684,.T.);
#9219=ORIENTED_EDGE('',*,*,#6685,.T.);
#9220=ORIENTED_EDGE('',*,*,#6686,.T.);
#9221=ORIENTED_EDGE('',*,*,#6682,.F.);
#9222=ORIENTED_EDGE('',*,*,#6687,.T.);
#9223=ORIENTED_EDGE('',*,*,#6688,.T.);
#9224=ORIENTED_EDGE('',*,*,#6689,.T.);
#9225=ORIENTED_EDGE('',*,*,#6685,.F.);
#9226=ORIENTED_EDGE('',*,*,#6690,.F.);
#9227=ORIENTED_EDGE('',*,*,#6691,.T.);
#9228=ORIENTED_EDGE('',*,*,#6692,.T.);
#9229=ORIENTED_EDGE('',*,*,#6688,.F.);
#9230=ORIENTED_EDGE('',*,*,#6693,.F.);
#9231=ORIENTED_EDGE('',*,*,#6559,.T.);
#9232=ORIENTED_EDGE('',*,*,#6694,.T.);
#9233=ORIENTED_EDGE('',*,*,#6695,.F.);
#9234=ORIENTED_EDGE('',*,*,#6696,.F.);
#9235=ORIENTED_EDGE('',*,*,#6695,.T.);
#9236=ORIENTED_EDGE('',*,*,#6697,.F.);
#9237=ORIENTED_EDGE('',*,*,#6698,.F.);
#9238=ORIENTED_EDGE('',*,*,#6699,.T.);
#9239=ORIENTED_EDGE('',*,*,#6690,.T.);
#9240=ORIENTED_EDGE('',*,*,#6687,.F.);
#9241=ORIENTED_EDGE('',*,*,#6684,.F.);
#9242=ORIENTED_EDGE('',*,*,#6681,.T.);
#9243=ORIENTED_EDGE('',*,*,#6678,.T.);
#9244=ORIENTED_EDGE('',*,*,#6582,.T.);
#9245=ORIENTED_EDGE('',*,*,#6587,.F.);
#9246=ORIENTED_EDGE('',*,*,#6583,.F.);
#9247=ORIENTED_EDGE('',*,*,#6619,.T.);
#9248=ORIENTED_EDGE('',*,*,#6616,.T.);
#9249=ORIENTED_EDGE('',*,*,#6613,.F.);
#9250=ORIENTED_EDGE('',*,*,#6610,.T.);
#9251=ORIENTED_EDGE('',*,*,#6607,.T.);
#9252=ORIENTED_EDGE('',*,*,#6604,.T.);
#9253=ORIENTED_EDGE('',*,*,#6601,.T.);
#9254=ORIENTED_EDGE('',*,*,#6598,.F.);
#9255=ORIENTED_EDGE('',*,*,#6595,.F.);
#9256=ORIENTED_EDGE('',*,*,#6592,.T.);
#9257=ORIENTED_EDGE('',*,*,#6589,.T.);
#9258=ORIENTED_EDGE('',*,*,#6573,.T.);
#9259=ORIENTED_EDGE('',*,*,#6642,.F.);
#9260=ORIENTED_EDGE('',*,*,#6638,.F.);
#9261=ORIENTED_EDGE('',*,*,#6674,.T.);
#9262=ORIENTED_EDGE('',*,*,#6671,.T.);
#9263=ORIENTED_EDGE('',*,*,#6668,.F.);
#9264=ORIENTED_EDGE('',*,*,#6665,.T.);
#9265=ORIENTED_EDGE('',*,*,#6662,.T.);
#9266=ORIENTED_EDGE('',*,*,#6659,.T.);
#9267=ORIENTED_EDGE('',*,*,#6656,.T.);
#9268=ORIENTED_EDGE('',*,*,#6653,.F.);
#9269=ORIENTED_EDGE('',*,*,#6650,.F.);
#9270=ORIENTED_EDGE('',*,*,#6647,.T.);
#9271=ORIENTED_EDGE('',*,*,#6644,.T.);
#9272=ORIENTED_EDGE('',*,*,#6571,.T.);
#9273=ORIENTED_EDGE('',*,*,#6625,.F.);
#9274=ORIENTED_EDGE('',*,*,#6621,.F.);
#9275=ORIENTED_EDGE('',*,*,#6636,.T.);
#9276=ORIENTED_EDGE('',*,*,#6633,.T.);
#9277=ORIENTED_EDGE('',*,*,#6629,.F.);
#9278=ORIENTED_EDGE('',*,*,#6700,.F.);
#9279=ORIENTED_EDGE('',*,*,#6701,.T.);
#9280=ORIENTED_EDGE('',*,*,#6702,.F.);
#9281=ORIENTED_EDGE('',*,*,#6703,.F.);
#9282=ORIENTED_EDGE('',*,*,#6704,.T.);
#9283=ORIENTED_EDGE('',*,*,#6705,.T.);
#9284=ORIENTED_EDGE('',*,*,#6706,.F.);
#9285=ORIENTED_EDGE('',*,*,#6707,.F.);
#9286=ORIENTED_EDGE('',*,*,#6708,.F.);
#9287=ORIENTED_EDGE('',*,*,#6709,.T.);
#9288=ORIENTED_EDGE('',*,*,#6710,.T.);
#9289=ORIENTED_EDGE('',*,*,#6711,.F.);
#9290=ORIENTED_EDGE('',*,*,#6712,.F.);
#9291=ORIENTED_EDGE('',*,*,#6713,.F.);
#9292=ORIENTED_EDGE('',*,*,#6714,.F.);
#9293=ORIENTED_EDGE('',*,*,#6715,.T.);
#9294=ORIENTED_EDGE('',*,*,#6716,.F.);
#9295=ORIENTED_EDGE('',*,*,#6717,.F.);
#9296=ORIENTED_EDGE('',*,*,#6718,.T.);
#9297=ORIENTED_EDGE('',*,*,#6719,.T.);
#9298=ORIENTED_EDGE('',*,*,#6720,.F.);
#9299=ORIENTED_EDGE('',*,*,#6721,.F.);
#9300=ORIENTED_EDGE('',*,*,#6722,.F.);
#9301=ORIENTED_EDGE('',*,*,#6723,.T.);
#9302=ORIENTED_EDGE('',*,*,#6724,.T.);
#9303=ORIENTED_EDGE('',*,*,#6725,.F.);
#9304=ORIENTED_EDGE('',*,*,#6726,.F.);
#9305=ORIENTED_EDGE('',*,*,#6727,.F.);
#9306=ORIENTED_EDGE('',*,*,#6728,.F.);
#9307=ORIENTED_EDGE('',*,*,#6729,.T.);
#9308=ORIENTED_EDGE('',*,*,#6730,.F.);
#9309=ORIENTED_EDGE('',*,*,#6731,.F.);
#9310=ORIENTED_EDGE('',*,*,#6732,.T.);
#9311=ORIENTED_EDGE('',*,*,#6733,.T.);
#9312=ORIENTED_EDGE('',*,*,#6734,.F.);
#9313=ORIENTED_EDGE('',*,*,#6735,.F.);
#9314=ORIENTED_EDGE('',*,*,#6736,.F.);
#9315=ORIENTED_EDGE('',*,*,#6737,.T.);
#9316=ORIENTED_EDGE('',*,*,#6738,.T.);
#9317=ORIENTED_EDGE('',*,*,#6739,.F.);
#9318=ORIENTED_EDGE('',*,*,#6693,.T.);
#9319=ORIENTED_EDGE('',*,*,#6696,.T.);
#9320=ORIENTED_EDGE('',*,*,#6740,.T.);
#9321=ORIENTED_EDGE('',*,*,#6741,.F.);
#9322=ORIENTED_EDGE('',*,*,#6742,.F.);
#9323=ORIENTED_EDGE('',*,*,#6743,.T.);
#9324=ORIENTED_EDGE('',*,*,#6744,.T.);
#9325=ORIENTED_EDGE('',*,*,#6560,.F.);
#9326=ORIENTED_EDGE('',*,*,#6627,.T.);
#9327=ORIENTED_EDGE('',*,*,#6565,.T.);
#9328=ORIENTED_EDGE('',*,*,#6676,.F.);
#9329=ORIENTED_EDGE('',*,*,#6556,.F.);
#9330=ORIENTED_EDGE('',*,*,#6578,.T.);
#9331=ORIENTED_EDGE('',*,*,#6745,.F.);
#9332=ORIENTED_EDGE('',*,*,#6744,.F.);
#9333=ORIENTED_EDGE('',*,*,#6746,.T.);
#9334=ORIENTED_EDGE('',*,*,#6747,.T.);
#9335=ORIENTED_EDGE('',*,*,#6561,.F.);
#9336=ORIENTED_EDGE('',*,*,#6743,.F.);
#9337=ORIENTED_EDGE('',*,*,#6748,.T.);
#9338=ORIENTED_EDGE('',*,*,#6749,.F.);
#9339=ORIENTED_EDGE('',*,*,#6746,.F.);
#9340=ORIENTED_EDGE('',*,*,#6750,.T.);
#9341=ORIENTED_EDGE('',*,*,#6751,.F.);
#9342=ORIENTED_EDGE('',*,*,#6752,.F.);
#9343=ORIENTED_EDGE('',*,*,#6741,.T.);
#9344=ORIENTED_EDGE('',*,*,#6753,.F.);
#9345=ORIENTED_EDGE('',*,*,#6706,.T.);
#9346=ORIENTED_EDGE('',*,*,#6754,.T.);
#9347=ORIENTED_EDGE('',*,*,#6755,.F.);
#9348=ORIENTED_EDGE('',*,*,#6756,.T.);
#9349=ORIENTED_EDGE('',*,*,#6757,.F.);
#9350=ORIENTED_EDGE('',*,*,#6758,.F.);
#9351=ORIENTED_EDGE('',*,*,#6720,.T.);
#9352=ORIENTED_EDGE('',*,*,#6745,.T.);
#9353=ORIENTED_EDGE('',*,*,#6759,.T.);
#9354=ORIENTED_EDGE('',*,*,#6760,.F.);
#9355=ORIENTED_EDGE('',*,*,#6759,.F.);
#9356=ORIENTED_EDGE('',*,*,#6761,.F.);
#9357=ORIENTED_EDGE('',*,*,#6734,.T.);
#9358=ORIENTED_EDGE('',*,*,#6762,.T.);
#9359=ORIENTED_EDGE('',*,*,#6763,.F.);
#9360=ORIENTED_EDGE('',*,*,#6732,.F.);
#9361=ORIENTED_EDGE('',*,*,#6764,.T.);
#9362=ORIENTED_EDGE('',*,*,#6765,.F.);
#9363=ORIENTED_EDGE('',*,*,#6766,.F.);
#9364=ORIENTED_EDGE('',*,*,#6733,.F.);
#9365=ORIENTED_EDGE('',*,*,#6766,.T.);
#9366=ORIENTED_EDGE('',*,*,#6767,.F.);
#9367=ORIENTED_EDGE('',*,*,#6762,.F.);
#9368=ORIENTED_EDGE('',*,*,#6721,.T.);
#9369=ORIENTED_EDGE('',*,*,#6758,.T.);
#9370=ORIENTED_EDGE('',*,*,#6768,.F.);
#9371=ORIENTED_EDGE('',*,*,#6769,.F.);
#9372=ORIENTED_EDGE('',*,*,#6722,.T.);
#9373=ORIENTED_EDGE('',*,*,#6769,.T.);
#9374=ORIENTED_EDGE('',*,*,#6770,.F.);
#9375=ORIENTED_EDGE('',*,*,#6771,.F.);
#9376=ORIENTED_EDGE('',*,*,#6723,.F.);
#9377=ORIENTED_EDGE('',*,*,#6771,.T.);
#9378=ORIENTED_EDGE('',*,*,#6772,.F.);
#9379=ORIENTED_EDGE('',*,*,#6773,.F.);
#9380=ORIENTED_EDGE('',*,*,#6724,.F.);
#9381=ORIENTED_EDGE('',*,*,#6773,.T.);
#9382=ORIENTED_EDGE('',*,*,#6774,.F.);
#9383=ORIENTED_EDGE('',*,*,#6775,.F.);
#9384=ORIENTED_EDGE('',*,*,#6725,.T.);
#9385=ORIENTED_EDGE('',*,*,#6775,.T.);
#9386=ORIENTED_EDGE('',*,*,#6776,.F.);
#9387=ORIENTED_EDGE('',*,*,#6777,.F.);
#9388=ORIENTED_EDGE('',*,*,#6726,.T.);
#9389=ORIENTED_EDGE('',*,*,#6777,.T.);
#9390=ORIENTED_EDGE('',*,*,#6778,.F.);
#9391=ORIENTED_EDGE('',*,*,#6779,.F.);
#9392=ORIENTED_EDGE('',*,*,#6727,.T.);
#9393=ORIENTED_EDGE('',*,*,#6779,.T.);
#9394=ORIENTED_EDGE('',*,*,#6780,.F.);
#9395=ORIENTED_EDGE('',*,*,#6781,.F.);
#9396=ORIENTED_EDGE('',*,*,#6728,.T.);
#9397=ORIENTED_EDGE('',*,*,#6781,.T.);
#9398=ORIENTED_EDGE('',*,*,#6782,.F.);
#9399=ORIENTED_EDGE('',*,*,#6783,.F.);
#9400=ORIENTED_EDGE('',*,*,#6729,.F.);
#9401=ORIENTED_EDGE('',*,*,#6783,.T.);
#9402=ORIENTED_EDGE('',*,*,#6784,.F.);
#9403=ORIENTED_EDGE('',*,*,#6785,.F.);
#9404=ORIENTED_EDGE('',*,*,#6730,.T.);
#9405=ORIENTED_EDGE('',*,*,#6785,.T.);
#9406=ORIENTED_EDGE('',*,*,#6786,.F.);
#9407=ORIENTED_EDGE('',*,*,#6787,.F.);
#9408=ORIENTED_EDGE('',*,*,#6731,.T.);
#9409=ORIENTED_EDGE('',*,*,#6787,.T.);
#9410=ORIENTED_EDGE('',*,*,#6788,.F.);
#9411=ORIENTED_EDGE('',*,*,#6764,.F.);
#9412=ORIENTED_EDGE('',*,*,#6704,.F.);
#9413=ORIENTED_EDGE('',*,*,#6789,.T.);
#9414=ORIENTED_EDGE('',*,*,#6790,.F.);
#9415=ORIENTED_EDGE('',*,*,#6791,.F.);
#9416=ORIENTED_EDGE('',*,*,#6705,.F.);
#9417=ORIENTED_EDGE('',*,*,#6791,.T.);
#9418=ORIENTED_EDGE('',*,*,#6792,.F.);
#9419=ORIENTED_EDGE('',*,*,#6754,.F.);
#9420=ORIENTED_EDGE('',*,*,#6742,.T.);
#9421=ORIENTED_EDGE('',*,*,#6752,.T.);
#9422=ORIENTED_EDGE('',*,*,#6793,.F.);
#9423=ORIENTED_EDGE('',*,*,#6748,.F.);
#9424=ORIENTED_EDGE('',*,*,#6700,.T.);
#9425=ORIENTED_EDGE('',*,*,#6632,.T.);
#9426=ORIENTED_EDGE('',*,*,#6794,.F.);
#9427=ORIENTED_EDGE('',*,*,#6795,.F.);
#9428=ORIENTED_EDGE('',*,*,#6701,.F.);
#9429=ORIENTED_EDGE('',*,*,#6795,.T.);
#9430=ORIENTED_EDGE('',*,*,#6796,.F.);
#9431=ORIENTED_EDGE('',*,*,#6797,.F.);
#9432=ORIENTED_EDGE('',*,*,#6702,.T.);
#9433=ORIENTED_EDGE('',*,*,#6797,.T.);
#9434=ORIENTED_EDGE('',*,*,#6798,.F.);
#9435=ORIENTED_EDGE('',*,*,#6799,.F.);
#9436=ORIENTED_EDGE('',*,*,#6703,.T.);
#9437=ORIENTED_EDGE('',*,*,#6799,.T.);
#9438=ORIENTED_EDGE('',*,*,#6800,.F.);
#9439=ORIENTED_EDGE('',*,*,#6789,.F.);
#9440=ORIENTED_EDGE('',*,*,#6718,.F.);
#9441=ORIENTED_EDGE('',*,*,#6801,.T.);
#9442=ORIENTED_EDGE('',*,*,#6802,.F.);
#9443=ORIENTED_EDGE('',*,*,#6803,.F.);
#9444=ORIENTED_EDGE('',*,*,#6719,.F.);
#9445=ORIENTED_EDGE('',*,*,#6803,.T.);
#9446=ORIENTED_EDGE('',*,*,#6804,.F.);
#9447=ORIENTED_EDGE('',*,*,#6756,.F.);
#9448=ORIENTED_EDGE('',*,*,#6707,.T.);
#9449=ORIENTED_EDGE('',*,*,#6753,.T.);
#9450=ORIENTED_EDGE('',*,*,#6805,.F.);
#9451=ORIENTED_EDGE('',*,*,#6806,.F.);
#9452=ORIENTED_EDGE('',*,*,#6708,.T.);
#9453=ORIENTED_EDGE('',*,*,#6806,.T.);
#9454=ORIENTED_EDGE('',*,*,#6807,.F.);
#9455=ORIENTED_EDGE('',*,*,#6808,.F.);
#9456=ORIENTED_EDGE('',*,*,#6709,.F.);
#9457=ORIENTED_EDGE('',*,*,#6808,.T.);
#9458=ORIENTED_EDGE('',*,*,#6809,.F.);
#9459=ORIENTED_EDGE('',*,*,#6810,.F.);
#9460=ORIENTED_EDGE('',*,*,#6710,.F.);
#9461=ORIENTED_EDGE('',*,*,#6810,.T.);
#9462=ORIENTED_EDGE('',*,*,#6811,.F.);
#9463=ORIENTED_EDGE('',*,*,#6812,.F.);
#9464=ORIENTED_EDGE('',*,*,#6711,.T.);
#9465=ORIENTED_EDGE('',*,*,#6812,.T.);
#9466=ORIENTED_EDGE('',*,*,#6813,.F.);
#9467=ORIENTED_EDGE('',*,*,#6814,.F.);
#9468=ORIENTED_EDGE('',*,*,#6712,.T.);
#9469=ORIENTED_EDGE('',*,*,#6814,.T.);
#9470=ORIENTED_EDGE('',*,*,#6815,.F.);
#9471=ORIENTED_EDGE('',*,*,#6816,.F.);
#9472=ORIENTED_EDGE('',*,*,#6713,.T.);
#9473=ORIENTED_EDGE('',*,*,#6816,.T.);
#9474=ORIENTED_EDGE('',*,*,#6817,.F.);
#9475=ORIENTED_EDGE('',*,*,#6818,.F.);
#9476=ORIENTED_EDGE('',*,*,#6714,.T.);
#9477=ORIENTED_EDGE('',*,*,#6818,.T.);
#9478=ORIENTED_EDGE('',*,*,#6819,.F.);
#9479=ORIENTED_EDGE('',*,*,#6820,.F.);
#9480=ORIENTED_EDGE('',*,*,#6715,.F.);
#9481=ORIENTED_EDGE('',*,*,#6820,.T.);
#9482=ORIENTED_EDGE('',*,*,#6821,.F.);
#9483=ORIENTED_EDGE('',*,*,#6822,.F.);
#9484=ORIENTED_EDGE('',*,*,#6716,.T.);
#9485=ORIENTED_EDGE('',*,*,#6822,.T.);
#9486=ORIENTED_EDGE('',*,*,#6823,.F.);
#9487=ORIENTED_EDGE('',*,*,#6824,.F.);
#9488=ORIENTED_EDGE('',*,*,#6717,.T.);
#9489=ORIENTED_EDGE('',*,*,#6824,.T.);
#9490=ORIENTED_EDGE('',*,*,#6825,.F.);
#9491=ORIENTED_EDGE('',*,*,#6801,.F.);
#9492=ORIENTED_EDGE('',*,*,#6740,.F.);
#9493=ORIENTED_EDGE('',*,*,#6698,.T.);
#9494=ORIENTED_EDGE('',*,*,#6826,.F.);
#9495=ORIENTED_EDGE('',*,*,#6750,.F.);
#9496=ORIENTED_EDGE('',*,*,#6735,.T.);
#9497=ORIENTED_EDGE('',*,*,#6761,.T.);
#9498=ORIENTED_EDGE('',*,*,#6827,.F.);
#9499=ORIENTED_EDGE('',*,*,#6828,.F.);
#9500=ORIENTED_EDGE('',*,*,#6736,.T.);
#9501=ORIENTED_EDGE('',*,*,#6828,.T.);
#9502=ORIENTED_EDGE('',*,*,#6829,.F.);
#9503=ORIENTED_EDGE('',*,*,#6830,.F.);
#9504=ORIENTED_EDGE('',*,*,#6737,.F.);
#9505=ORIENTED_EDGE('',*,*,#6830,.T.);
#9506=ORIENTED_EDGE('',*,*,#6831,.F.);
#9507=ORIENTED_EDGE('',*,*,#6832,.F.);
#9508=ORIENTED_EDGE('',*,*,#6738,.F.);
#9509=ORIENTED_EDGE('',*,*,#6832,.T.);
#9510=ORIENTED_EDGE('',*,*,#6833,.F.);
#9511=ORIENTED_EDGE('',*,*,#6834,.F.);
#9512=ORIENTED_EDGE('',*,*,#6739,.T.);
#9513=ORIENTED_EDGE('',*,*,#6834,.T.);
#9514=ORIENTED_EDGE('',*,*,#6835,.F.);
#9515=ORIENTED_EDGE('',*,*,#6836,.F.);
#9516=ORIENTED_EDGE('',*,*,#6699,.F.);
#9517=ORIENTED_EDGE('',*,*,#6836,.T.);
#9518=ORIENTED_EDGE('',*,*,#6837,.T.);
#9519=ORIENTED_EDGE('',*,*,#6691,.F.);
#9520=ORIENTED_EDGE('',*,*,#6837,.F.);
#9521=ORIENTED_EDGE('',*,*,#6835,.T.);
#9522=ORIENTED_EDGE('',*,*,#6833,.T.);
#9523=ORIENTED_EDGE('',*,*,#6831,.T.);
#9524=ORIENTED_EDGE('',*,*,#6829,.T.);
#9525=ORIENTED_EDGE('',*,*,#6827,.T.);
#9526=ORIENTED_EDGE('',*,*,#6763,.T.);
#9527=ORIENTED_EDGE('',*,*,#6767,.T.);
#9528=ORIENTED_EDGE('',*,*,#6765,.T.);
#9529=ORIENTED_EDGE('',*,*,#6788,.T.);
#9530=ORIENTED_EDGE('',*,*,#6786,.T.);
#9531=ORIENTED_EDGE('',*,*,#6784,.T.);
#9532=ORIENTED_EDGE('',*,*,#6782,.T.);
#9533=ORIENTED_EDGE('',*,*,#6780,.T.);
#9534=ORIENTED_EDGE('',*,*,#6778,.T.);
#9535=ORIENTED_EDGE('',*,*,#6776,.T.);
#9536=ORIENTED_EDGE('',*,*,#6774,.T.);
#9537=ORIENTED_EDGE('',*,*,#6772,.T.);
#9538=ORIENTED_EDGE('',*,*,#6770,.T.);
#9539=ORIENTED_EDGE('',*,*,#6768,.T.);
#9540=ORIENTED_EDGE('',*,*,#6757,.T.);
#9541=ORIENTED_EDGE('',*,*,#6804,.T.);
#9542=ORIENTED_EDGE('',*,*,#6802,.T.);
#9543=ORIENTED_EDGE('',*,*,#6825,.T.);
#9544=ORIENTED_EDGE('',*,*,#6823,.T.);
#9545=ORIENTED_EDGE('',*,*,#6821,.T.);
#9546=ORIENTED_EDGE('',*,*,#6819,.T.);
#9547=ORIENTED_EDGE('',*,*,#6817,.T.);
#9548=ORIENTED_EDGE('',*,*,#6815,.T.);
#9549=ORIENTED_EDGE('',*,*,#6813,.T.);
#9550=ORIENTED_EDGE('',*,*,#6811,.T.);
#9551=ORIENTED_EDGE('',*,*,#6809,.T.);
#9552=ORIENTED_EDGE('',*,*,#6807,.T.);
#9553=ORIENTED_EDGE('',*,*,#6805,.T.);
#9554=ORIENTED_EDGE('',*,*,#6755,.T.);
#9555=ORIENTED_EDGE('',*,*,#6792,.T.);
#9556=ORIENTED_EDGE('',*,*,#6790,.T.);
#9557=ORIENTED_EDGE('',*,*,#6800,.T.);
#9558=ORIENTED_EDGE('',*,*,#6798,.T.);
#9559=ORIENTED_EDGE('',*,*,#6796,.T.);
#9560=ORIENTED_EDGE('',*,*,#6794,.T.);
#9561=ORIENTED_EDGE('',*,*,#6631,.F.);
#9562=ORIENTED_EDGE('',*,*,#6635,.F.);
#9563=ORIENTED_EDGE('',*,*,#6637,.F.);
#9564=ORIENTED_EDGE('',*,*,#6623,.F.);
#9565=ORIENTED_EDGE('',*,*,#6626,.F.);
#9566=ORIENTED_EDGE('',*,*,#6569,.F.);
#9567=ORIENTED_EDGE('',*,*,#6646,.F.);
#9568=ORIENTED_EDGE('',*,*,#6649,.F.);
#9569=ORIENTED_EDGE('',*,*,#6652,.F.);
#9570=ORIENTED_EDGE('',*,*,#6655,.F.);
#9571=ORIENTED_EDGE('',*,*,#6658,.F.);
#9572=ORIENTED_EDGE('',*,*,#6661,.F.);
#9573=ORIENTED_EDGE('',*,*,#6664,.F.);
#9574=ORIENTED_EDGE('',*,*,#6667,.F.);
#9575=ORIENTED_EDGE('',*,*,#6670,.F.);
#9576=ORIENTED_EDGE('',*,*,#6673,.F.);
#9577=ORIENTED_EDGE('',*,*,#6675,.F.);
#9578=ORIENTED_EDGE('',*,*,#6640,.F.);
#9579=ORIENTED_EDGE('',*,*,#6643,.F.);
#9580=ORIENTED_EDGE('',*,*,#6575,.F.);
#9581=ORIENTED_EDGE('',*,*,#6591,.F.);
#9582=ORIENTED_EDGE('',*,*,#6594,.F.);
#9583=ORIENTED_EDGE('',*,*,#6597,.F.);
#9584=ORIENTED_EDGE('',*,*,#6600,.F.);
#9585=ORIENTED_EDGE('',*,*,#6603,.F.);
#9586=ORIENTED_EDGE('',*,*,#6606,.F.);
#9587=ORIENTED_EDGE('',*,*,#6609,.F.);
#9588=ORIENTED_EDGE('',*,*,#6612,.F.);
#9589=ORIENTED_EDGE('',*,*,#6615,.F.);
#9590=ORIENTED_EDGE('',*,*,#6618,.F.);
#9591=ORIENTED_EDGE('',*,*,#6620,.F.);
#9592=ORIENTED_EDGE('',*,*,#6585,.F.);
#9593=ORIENTED_EDGE('',*,*,#6588,.F.);
#9594=ORIENTED_EDGE('',*,*,#6580,.F.);
#9595=ORIENTED_EDGE('',*,*,#6680,.F.);
#9596=ORIENTED_EDGE('',*,*,#6683,.F.);
#9597=ORIENTED_EDGE('',*,*,#6686,.F.);
#9598=ORIENTED_EDGE('',*,*,#6689,.F.);
#9599=ORIENTED_EDGE('',*,*,#6692,.F.);
#9600=ORIENTED_EDGE('',*,*,#6576,.F.);
#9601=ORIENTED_EDGE('',*,*,#6694,.F.);
#9602=ORIENTED_EDGE('',*,*,#6558,.F.);
#9603=ORIENTED_EDGE('',*,*,#6677,.F.);
#9604=ORIENTED_EDGE('',*,*,#6567,.F.);
#9605=ORIENTED_EDGE('',*,*,#6628,.F.);
#9606=ORIENTED_EDGE('',*,*,#6562,.F.);
#9607=ORIENTED_EDGE('',*,*,#6747,.F.);
#9608=ORIENTED_EDGE('',*,*,#6749,.T.);
#9609=ORIENTED_EDGE('',*,*,#6793,.T.);
#9610=ORIENTED_EDGE('',*,*,#6751,.T.);
#9611=ORIENTED_EDGE('',*,*,#6826,.T.);
#9612=ORIENTED_EDGE('',*,*,#6697,.T.);
#9613=ORIENTED_EDGE('',*,*,#6760,.T.);
#10573=CYLINDRICAL_SURFACE('',#12015,2.1);
#10574=CYLINDRICAL_SURFACE('',#12027,0.500000000000003);
#10575=CYLINDRICAL_SURFACE('',#12048,0.500000000000003);
#10576=CYLINDRICAL_SURFACE('',#12072,2.1);
#10577=CYLINDRICAL_SURFACE('',#12083,0.500000000000003);
#10578=CYLINDRICAL_SURFACE('',#12104,0.500000000000003);
#11010=ADVANCED_FACE('',(#1389),#540,.F.);
#11011=ADVANCED_FACE('',(#1390),#541,.T.);
#11012=ADVANCED_FACE('',(#1391),#542,.F.);
#11013=ADVANCED_FACE('',(#1392),#543,.F.);
#11014=ADVANCED_FACE('',(#1393),#544,.F.);
#11015=ADVANCED_FACE('',(#1394),#10573,.F.);
#11016=ADVANCED_FACE('',(#1395),#545,.F.);
#11017=ADVANCED_FACE('',(#1396),#546,.F.);
#11018=ADVANCED_FACE('',(#1397),#547,.F.);
#11019=ADVANCED_FACE('',(#1398),#548,.F.);
#11020=ADVANCED_FACE('',(#1399),#549,.F.);
#11021=ADVANCED_FACE('',(#1400),#550,.F.);
#11022=ADVANCED_FACE('',(#1401),#551,.F.);
#11023=ADVANCED_FACE('',(#1402),#552,.F.);
#11024=ADVANCED_FACE('',(#1403),#553,.F.);
#11025=ADVANCED_FACE('',(#1404),#10574,.T.);
#11026=ADVANCED_FACE('',(#1405),#554,.F.);
#11027=ADVANCED_FACE('',(#1406),#555,.F.);
#11028=ADVANCED_FACE('',(#1407),#556,.F.);
#11029=ADVANCED_FACE('',(#1408),#557,.F.);
#11030=ADVANCED_FACE('',(#1409),#558,.F.);
#11031=ADVANCED_FACE('',(#1410),#559,.F.);
#11032=ADVANCED_FACE('',(#1411),#560,.F.);
#11033=ADVANCED_FACE('',(#1412),#561,.F.);
#11034=ADVANCED_FACE('',(#1413),#562,.F.);
#11035=ADVANCED_FACE('',(#1414),#563,.F.);
#11036=ADVANCED_FACE('',(#1415),#564,.F.);
#11037=ADVANCED_FACE('',(#1416),#565,.F.);
#11038=ADVANCED_FACE('',(#1417),#566,.F.);
#11039=ADVANCED_FACE('',(#1418),#567,.F.);
#11040=ADVANCED_FACE('',(#1419),#568,.F.);
#11041=ADVANCED_FACE('',(#1420),#569,.F.);
#11042=ADVANCED_FACE('',(#1421),#570,.F.);
#11043=ADVANCED_FACE('',(#1422),#571,.F.);
#11044=ADVANCED_FACE('',(#1423),#10575,.T.);
#11045=ADVANCED_FACE('',(#1424),#572,.F.);
#11046=ADVANCED_FACE('',(#1425),#573,.F.);
#11047=ADVANCED_FACE('',(#1426),#574,.F.);
#11048=ADVANCED_FACE('',(#1427),#575,.F.);
#11049=ADVANCED_FACE('',(#1428),#576,.F.);
#11050=ADVANCED_FACE('',(#1429),#577,.F.);
#11051=ADVANCED_FACE('',(#1430),#578,.F.);
#11052=ADVANCED_FACE('',(#1431),#579,.F.);
#11053=ADVANCED_FACE('',(#1432),#580,.F.);
#11054=ADVANCED_FACE('',(#1433),#581,.F.);
#11055=ADVANCED_FACE('',(#1434),#582,.T.);
#11056=ADVANCED_FACE('',(#1435),#583,.T.);
#11057=ADVANCED_FACE('',(#1436,#172,#173,#174),#584,.F.);
#11058=ADVANCED_FACE('',(#1437),#585,.F.);
#11059=ADVANCED_FACE('',(#1438),#586,.F.);
#11060=ADVANCED_FACE('',(#1439),#587,.T.);
#11061=ADVANCED_FACE('',(#1440),#588,.T.);
#11062=ADVANCED_FACE('',(#1441),#589,.T.);
#11063=ADVANCED_FACE('',(#1442),#10576,.F.);
#11064=ADVANCED_FACE('',(#1443),#590,.T.);
#11065=ADVANCED_FACE('',(#1444),#591,.T.);
#11066=ADVANCED_FACE('',(#1445),#592,.T.);
#11067=ADVANCED_FACE('',(#1446),#593,.T.);
#11068=ADVANCED_FACE('',(#1447),#594,.T.);
#11069=ADVANCED_FACE('',(#1448),#595,.T.);
#11070=ADVANCED_FACE('',(#1449),#596,.T.);
#11071=ADVANCED_FACE('',(#1450),#597,.T.);
#11072=ADVANCED_FACE('',(#1451),#598,.T.);
#11073=ADVANCED_FACE('',(#1452),#10577,.T.);
#11074=ADVANCED_FACE('',(#1453),#599,.T.);
#11075=ADVANCED_FACE('',(#1454),#600,.T.);
#11076=ADVANCED_FACE('',(#1455),#601,.T.);
#11077=ADVANCED_FACE('',(#1456),#602,.T.);
#11078=ADVANCED_FACE('',(#1457),#603,.T.);
#11079=ADVANCED_FACE('',(#1458),#604,.T.);
#11080=ADVANCED_FACE('',(#1459),#605,.T.);
#11081=ADVANCED_FACE('',(#1460),#606,.T.);
#11082=ADVANCED_FACE('',(#1461),#607,.T.);
#11083=ADVANCED_FACE('',(#1462),#608,.T.);
#11084=ADVANCED_FACE('',(#1463),#609,.T.);
#11085=ADVANCED_FACE('',(#1464),#610,.T.);
#11086=ADVANCED_FACE('',(#1465),#611,.T.);
#11087=ADVANCED_FACE('',(#1466),#612,.T.);
#11088=ADVANCED_FACE('',(#1467),#613,.T.);
#11089=ADVANCED_FACE('',(#1468),#614,.T.);
#11090=ADVANCED_FACE('',(#1469),#615,.T.);
#11091=ADVANCED_FACE('',(#1470),#616,.T.);
#11092=ADVANCED_FACE('',(#1471),#617,.T.);
#11093=ADVANCED_FACE('',(#1472),#10578,.T.);
#11094=ADVANCED_FACE('',(#1473),#618,.T.);
#11095=ADVANCED_FACE('',(#1474),#619,.T.);
#11096=ADVANCED_FACE('',(#1475),#620,.T.);
#11097=ADVANCED_FACE('',(#1476),#621,.T.);
#11098=ADVANCED_FACE('',(#1477),#622,.T.);
#11099=ADVANCED_FACE('',(#1478),#623,.T.);
#11100=ADVANCED_FACE('',(#1479),#624,.T.);
#11101=ADVANCED_FACE('',(#1480),#625,.T.);
#11102=ADVANCED_FACE('',(#1481),#626,.T.);
#11103=ADVANCED_FACE('',(#1482),#627,.T.);
#11104=ADVANCED_FACE('',(#1483),#628,.T.);
#11105=ADVANCED_FACE('',(#1484,#175,#176,#177),#629,.T.);
#11286=CLOSED_SHELL('',(#11010,#11011,#11012,#11013,#11014,#11015,#11016,
#11017,#11018,#11019,#11020,#11021,#11022,#11023,#11024,#11025,#11026,#11027,
#11028,#11029,#11030,#11031,#11032,#11033,#11034,#11035,#11036,#11037,#11038,
#11039,#11040,#11041,#11042,#11043,#11044,#11045,#11046,#11047,#11048,#11049,
#11050,#11051,#11052,#11053,#11054,#11055,#11056,#11057,#11058,#11059,#11060,
#11061,#11062,#11063,#11064,#11065,#11066,#11067,#11068,#11069,#11070,#11071,
#11072,#11073,#11074,#11075,#11076,#11077,#11078,#11079,#11080,#11081,#11082,
#11083,#11084,#11085,#11086,#11087,#11088,#11089,#11090,#11091,#11092,#11093,
#11094,#11095,#11096,#11097,#11098,#11099,#11100,#11101,#11102,#11103,#11104,
#11105));
#12009=AXIS2_PLACEMENT_3D('',#34884,#14003,#14004);
#12010=AXIS2_PLACEMENT_3D('',#34885,#14005,#14006);
#12011=AXIS2_PLACEMENT_3D('',#34894,#14011,#14012);
#12012=AXIS2_PLACEMENT_3D('',#34903,#14017,#14018);
#12013=AXIS2_PLACEMENT_3D('',#34912,#14023,#14024);
#12014=AXIS2_PLACEMENT_3D('',#34921,#14029,#14030);
#12015=AXIS2_PLACEMENT_3D('',#34930,#14035,#14036);
#12016=AXIS2_PLACEMENT_3D('',#34932,#14037,#14038);
#12017=AXIS2_PLACEMENT_3D('',#34935,#14040,#14041);
#12018=AXIS2_PLACEMENT_3D('',#34936,#14042,#14043);
#12019=AXIS2_PLACEMENT_3D('',#34945,#14048,#14049);
#12020=AXIS2_PLACEMENT_3D('',#34954,#14054,#14055);
#12021=AXIS2_PLACEMENT_3D('',#34957,#14058,#14059);
#12022=AXIS2_PLACEMENT_3D('',#34963,#14063,#14064);
#12023=AXIS2_PLACEMENT_3D('',#34969,#14068,#14069);
#12024=AXIS2_PLACEMENT_3D('',#34975,#14073,#14074);
#12025=AXIS2_PLACEMENT_3D('',#34981,#14078,#14079);
#12026=AXIS2_PLACEMENT_3D('',#34987,#14083,#14084);
#12027=AXIS2_PLACEMENT_3D('',#34993,#14088,#14089);
#12028=AXIS2_PLACEMENT_3D('',#34995,#14090,#14091);
#12029=AXIS2_PLACEMENT_3D('',#34998,#14093,#14094);
#12030=AXIS2_PLACEMENT_3D('',#34999,#14095,#14096);
#12031=AXIS2_PLACEMENT_3D('',#35005,#14100,#14101);
#12032=AXIS2_PLACEMENT_3D('',#35011,#14105,#14106);
#12033=AXIS2_PLACEMENT_3D('',#35017,#14110,#14111);
#12034=AXIS2_PLACEMENT_3D('',#35020,#14114,#14115);
#12035=AXIS2_PLACEMENT_3D('',#35029,#14120,#14121);
#12036=AXIS2_PLACEMENT_3D('',#35032,#14124,#14125);
#12037=AXIS2_PLACEMENT_3D('',#35035,#14128,#14129);
#12038=AXIS2_PLACEMENT_3D('',#35044,#14134,#14135);
#12039=AXIS2_PLACEMENT_3D('',#35050,#14139,#14140);
#12040=AXIS2_PLACEMENT_3D('',#35053,#14143,#14144);
#12041=AXIS2_PLACEMENT_3D('',#35062,#14149,#14150);
#12042=AXIS2_PLACEMENT_3D('',#35065,#14153,#14154);
#12043=AXIS2_PLACEMENT_3D('',#35071,#14158,#14159);
#12044=AXIS2_PLACEMENT_3D('',#35077,#14163,#14164);
#12045=AXIS2_PLACEMENT_3D('',#35083,#14168,#14169);
#12046=AXIS2_PLACEMENT_3D('',#35089,#14173,#14174);
#12047=AXIS2_PLACEMENT_3D('',#35095,#14178,#14179);
#12048=AXIS2_PLACEMENT_3D('',#35101,#14183,#14184);
#12049=AXIS2_PLACEMENT_3D('',#35103,#14185,#14186);
#12050=AXIS2_PLACEMENT_3D('',#35106,#14188,#14189);
#12051=AXIS2_PLACEMENT_3D('',#35107,#14190,#14191);
#12052=AXIS2_PLACEMENT_3D('',#35113,#14195,#14196);
#12053=AXIS2_PLACEMENT_3D('',#35119,#14200,#14201);
#12054=AXIS2_PLACEMENT_3D('',#35125,#14205,#14206);
#12055=AXIS2_PLACEMENT_3D('',#35128,#14209,#14210);
#12056=AXIS2_PLACEMENT_3D('',#35131,#14213,#14214);
#12057=AXIS2_PLACEMENT_3D('',#35137,#14218,#14219);
#12058=AXIS2_PLACEMENT_3D('',#35143,#14223,#14224);
#12059=AXIS2_PLACEMENT_3D('',#35149,#14228,#14229);
#12060=AXIS2_PLACEMENT_3D('',#35155,#14233,#14234);
#12061=AXIS2_PLACEMENT_3D('',#35161,#14238,#14239);
#12062=AXIS2_PLACEMENT_3D('',#35167,#14243,#14244);
#12063=AXIS2_PLACEMENT_3D('',#35173,#14248,#14249);
#12064=AXIS2_PLACEMENT_3D('',#35203,#14264,#14265);
#12065=AXIS2_PLACEMENT_3D('',#35231,#14279,#14280);
#12066=AXIS2_PLACEMENT_3D('',#35265,#14298,#14299);
#12067=AXIS2_PLACEMENT_3D('',#35266,#14300,#14301);
#12068=AXIS2_PLACEMENT_3D('',#35270,#14304,#14305);
#12069=AXIS2_PLACEMENT_3D('',#35274,#14308,#14309);
#12070=AXIS2_PLACEMENT_3D('',#35280,#14313,#14314);
#12071=AXIS2_PLACEMENT_3D('',#35286,#14318,#14319);
#12072=AXIS2_PLACEMENT_3D('',#35292,#14323,#14324);
#12073=AXIS2_PLACEMENT_3D('',#35295,#14326,#14327);
#12074=AXIS2_PLACEMENT_3D('',#35296,#14328,#14329);
#12075=AXIS2_PLACEMENT_3D('',#35302,#14333,#14334);
#12076=AXIS2_PLACEMENT_3D('',#35308,#14338,#14339);
#12077=AXIS2_PLACEMENT_3D('',#35310,#14341,#14342);
#12078=AXIS2_PLACEMENT_3D('',#35314,#14345,#14346);
#12079=AXIS2_PLACEMENT_3D('',#35318,#14349,#14350);
#12080=AXIS2_PLACEMENT_3D('',#35322,#14353,#14354);
#12081=AXIS2_PLACEMENT_3D('',#35326,#14357,#14358);
#12082=AXIS2_PLACEMENT_3D('',#35330,#14361,#14362);
#12083=AXIS2_PLACEMENT_3D('',#35334,#14365,#14366);
#12084=AXIS2_PLACEMENT_3D('',#35336,#14367,#14368);
#12085=AXIS2_PLACEMENT_3D('',#35338,#14370,#14371);
#12086=AXIS2_PLACEMENT_3D('',#35342,#14374,#14375);
#12087=AXIS2_PLACEMENT_3D('',#35346,#14378,#14379);
#12088=AXIS2_PLACEMENT_3D('',#35350,#14382,#14383);
#12089=AXIS2_PLACEMENT_3D('',#35352,#14385,#14386);
#12090=AXIS2_PLACEMENT_3D('',#35358,#14390,#14391);
#12091=AXIS2_PLACEMENT_3D('',#35360,#14393,#14394);
#12092=AXIS2_PLACEMENT_3D('',#35362,#14396,#14397);
#12093=AXIS2_PLACEMENT_3D('',#35366,#14400,#14401);
#12094=AXIS2_PLACEMENT_3D('',#35370,#14404,#14405);
#12095=AXIS2_PLACEMENT_3D('',#35374,#14408,#14409);
#12096=AXIS2_PLACEMENT_3D('',#35376,#14411,#14412);
#12097=AXIS2_PLACEMENT_3D('',#35382,#14416,#14417);
#12098=AXIS2_PLACEMENT_3D('',#35384,#14419,#14420);
#12099=AXIS2_PLACEMENT_3D('',#35388,#14423,#14424);
#12100=AXIS2_PLACEMENT_3D('',#35392,#14427,#14428);
#12101=AXIS2_PLACEMENT_3D('',#35396,#14431,#14432);
#12102=AXIS2_PLACEMENT_3D('',#35400,#14435,#14436);
#12103=AXIS2_PLACEMENT_3D('',#35404,#14439,#14440);
#12104=AXIS2_PLACEMENT_3D('',#35408,#14443,#14444);
#12105=AXIS2_PLACEMENT_3D('',#35410,#14445,#14446);
#12106=AXIS2_PLACEMENT_3D('',#35412,#14448,#14449);
#12107=AXIS2_PLACEMENT_3D('',#35416,#14452,#14453);
#12108=AXIS2_PLACEMENT_3D('',#35420,#14456,#14457);
#12109=AXIS2_PLACEMENT_3D('',#35424,#14460,#14461);
#12110=AXIS2_PLACEMENT_3D('',#35426,#14463,#14464);
#12111=AXIS2_PLACEMENT_3D('',#35428,#14466,#14467);
#12112=AXIS2_PLACEMENT_3D('',#35432,#14470,#14471);
#12113=AXIS2_PLACEMENT_3D('',#35436,#14474,#14475);
#12114=AXIS2_PLACEMENT_3D('',#35440,#14478,#14479);
#12115=AXIS2_PLACEMENT_3D('',#35444,#14482,#14483);
#12116=AXIS2_PLACEMENT_3D('',#35448,#14486,#14487);
#12117=AXIS2_PLACEMENT_3D('',#35450,#14489,#14490);
#14003=DIRECTION('axis',(0.,0.,1.));
#14004=DIRECTION('refdir',(1.,0.,0.));
#14005=DIRECTION('center_axis',(1.,0.,1.02489030670754E-15));
#14006=DIRECTION('ref_axis',(1.02489030670754E-15,0.,-1.));
#14007=DIRECTION('',(-1.02489030670754E-15,0.,1.));
#14008=DIRECTION('',(0.,1.,0.));
#14009=DIRECTION('',(1.02489030670754E-15,0.,-1.));
#14010=DIRECTION('',(0.,1.,0.));
#14011=DIRECTION('center_axis',(-1.,0.,-1.02489030670754E-15));
#14012=DIRECTION('ref_axis',(-1.02489030670754E-15,0.,1.));
#14013=DIRECTION('',(-1.02489030670754E-15,0.,1.));
#14014=DIRECTION('',(0.,1.,0.));
#14015=DIRECTION('',(1.02489030670754E-15,0.,-1.));
#14016=DIRECTION('',(0.,1.,0.));
#14017=DIRECTION('center_axis',(1.,0.,1.02489030670754E-15));
#14018=DIRECTION('ref_axis',(1.02489030670754E-15,0.,-1.));
#14019=DIRECTION('',(0.,1.,0.));
#14020=DIRECTION('',(1.02489030670754E-15,0.,-1.));
#14021=DIRECTION('',(0.,1.,0.));
#14022=DIRECTION('',(-1.02489030670754E-15,0.,1.));
#14023=DIRECTION('center_axis',(1.02489030670754E-15,0.,-1.));
#14024=DIRECTION('ref_axis',(-1.,0.,-1.02489030670754E-15));
#14025=DIRECTION('',(0.,1.,0.));
#14026=DIRECTION('',(1.,0.,1.02489030670754E-15));
#14027=DIRECTION('',(0.,1.,0.));
#14028=DIRECTION('',(-1.,0.,-1.02489030670754E-15));
#14029=DIRECTION('center_axis',(-1.,0.,-1.02489030670754E-15));
#14030=DIRECTION('ref_axis',(-1.02489030670754E-15,0.,1.));
#14031=DIRECTION('',(0.,1.,0.));
#14032=DIRECTION('',(-1.02489030670754E-15,0.,1.));
#14033=DIRECTION('',(0.,1.,0.));
#14034=DIRECTION('',(1.02489030670754E-15,0.,-1.));
#14035=DIRECTION('center_axis',(0.,-1.,0.));
#14036=DIRECTION('ref_axis',(-1.,0.,-1.02489030670754E-15));
#14037=DIRECTION('center_axis',(0.,-1.,0.));
#14038=DIRECTION('ref_axis',(-1.,0.,-1.02489030670754E-15));
#14039=DIRECTION('',(0.,-1.,0.));
#14040=DIRECTION('center_axis',(0.,1.,0.));
#14041=DIRECTION('ref_axis',(-1.,0.,-1.02489030670754E-15));
#14042=DIRECTION('center_axis',(-1.02489030670754E-15,0.,1.));
#14043=DIRECTION('ref_axis',(1.,0.,1.02489030670754E-15));
#14044=DIRECTION('',(0.,1.,0.));
#14045=DIRECTION('',(-1.,0.,-1.02489030670754E-15));
#14046=DIRECTION('',(0.,1.,0.));
#14047=DIRECTION('',(1.,0.,1.02489030670754E-15));
#14048=DIRECTION('center_axis',(1.,0.,8.41193286835436E-16));
#14049=DIRECTION('ref_axis',(8.41193286835436E-16,0.,-1.));
#14050=DIRECTION('',(-8.41193286835436E-16,0.,1.));
#14051=DIRECTION('',(0.,1.,0.));
#14052=DIRECTION('',(-8.41193286835436E-16,0.,1.));
#14053=DIRECTION('',(0.,1.,0.));
#14054=DIRECTION('center_axis',(0.707106781186547,0.,0.707106781186548));
#14055=DIRECTION('ref_axis',(0.707106781186548,0.,-0.707106781186547));
#14056=DIRECTION('',(-0.707106781186548,0.,0.707106781186547));
#14057=DIRECTION('',(-0.707106781186548,0.,0.707106781186547));
#14058=DIRECTION('center_axis',(-0.707106781186547,0.,-0.707106781186548));
#14059=DIRECTION('ref_axis',(-0.707106781186548,0.,0.707106781186547));
#14060=DIRECTION('',(-0.707106781186548,0.,0.707106781186547));
#14061=DIRECTION('',(0.,1.,0.));
#14062=DIRECTION('',(0.707106781186548,0.,-0.707106781186547));
#14063=DIRECTION('center_axis',(-5.24835571952591E-16,0.,-1.));
#14064=DIRECTION('ref_axis',(-1.,0.,5.24835571952591E-16));
#14065=DIRECTION('',(-1.,0.,5.24835571952591E-16));
#14066=DIRECTION('',(0.,1.,0.));
#14067=DIRECTION('',(1.,0.,-5.24835571952591E-16));
#14068=DIRECTION('center_axis',(1.,0.,-8.04181361684024E-17));
#14069=DIRECTION('ref_axis',(-8.04181361684024E-17,0.,-1.));
#14070=DIRECTION('',(8.04181361684024E-17,0.,1.));
#14071=DIRECTION('',(0.,1.,0.));
#14072=DIRECTION('',(8.04181361684024E-17,0.,1.));
#14073=DIRECTION('center_axis',(8.41193286835436E-16,0.,-1.));
#14074=DIRECTION('ref_axis',(-1.,0.,-8.41193286835436E-16));
#14075=DIRECTION('',(1.,0.,8.41193286835436E-16));
#14076=DIRECTION('',(0.,1.,0.));
#14077=DIRECTION('',(1.,0.,8.41193286835436E-16));
#14078=DIRECTION('center_axis',(-0.707106781186547,0.,-0.707106781186548));
#14079=DIRECTION('ref_axis',(-0.707106781186548,0.,0.707106781186547));
#14080=DIRECTION('',(-0.707106781186548,0.,0.707106781186547));
#14081=DIRECTION('',(0.,1.,0.));
#14082=DIRECTION('',(0.707106781186548,0.,-0.707106781186547));
#14083=DIRECTION('center_axis',(-1.,0.,-3.89980473439034E-16));
#14084=DIRECTION('ref_axis',(-3.89980473439034E-16,0.,1.));
#14085=DIRECTION('',(-3.89980473439034E-16,0.,1.));
#14086=DIRECTION('',(0.,1.,0.));
#14087=DIRECTION('',(3.89980473439034E-16,0.,-1.));
#14088=DIRECTION('center_axis',(0.,-1.,0.));
#14089=DIRECTION('ref_axis',(7.50253143458634E-15,0.,-1.));
#14090=DIRECTION('center_axis',(0.,-1.,0.));
#14091=DIRECTION('ref_axis',(7.50253143458634E-15,0.,-1.));
#14092=DIRECTION('',(0.,1.,0.));
#14093=DIRECTION('center_axis',(0.,1.,0.));
#14094=DIRECTION('ref_axis',(7.50253143458634E-15,0.,-1.));
#14095=DIRECTION('center_axis',(-8.41193286835436E-16,0.,1.));
#14096=DIRECTION('ref_axis',(1.,0.,8.41193286835436E-16));
#14097=DIRECTION('',(1.,0.,8.41193286835436E-16));
#14098=DIRECTION('',(0.,1.,0.));
#14099=DIRECTION('',(-1.,0.,-8.41193286835436E-16));
#14100=DIRECTION('center_axis',(0.707106781186546,0.,0.707106781186549));
#14101=DIRECTION('ref_axis',(0.707106781186549,0.,-0.707106781186546));
#14102=DIRECTION('',(-0.707106781186549,0.,0.707106781186546));
#14103=DIRECTION('',(0.,1.,0.));
#14104=DIRECTION('',(-0.707106781186549,0.,0.707106781186546));
#14105=DIRECTION('center_axis',(1.,0.,8.41193286835436E-16));
#14106=DIRECTION('ref_axis',(8.41193286835436E-16,0.,-1.));
#14107=DIRECTION('',(8.41193286835436E-16,0.,-1.));
#14108=DIRECTION('',(0.,1.,0.));
#14109=DIRECTION('',(-8.41193286835436E-16,0.,1.));
#14110=DIRECTION('center_axis',(8.41193286835436E-16,0.,-1.));
#14111=DIRECTION('ref_axis',(-1.,0.,-8.41193286835436E-16));
#14112=DIRECTION('',(-1.,0.,-8.41193286835436E-16));
#14113=DIRECTION('',(1.,0.,8.41193286835436E-16));
#14114=DIRECTION('center_axis',(-1.,0.,-9.63657966750171E-16));
#14115=DIRECTION('ref_axis',(-9.63657966750171E-16,0.,1.));
#14116=DIRECTION('',(9.63657966750171E-16,0.,-1.));
#14117=DIRECTION('',(0.,1.,0.));
#14118=DIRECTION('',(9.63657966750171E-16,0.,-1.));
#14119=DIRECTION('',(0.,1.,0.));
#14120=DIRECTION('center_axis',(-0.707106781186547,0.,-0.707106781186548));
#14121=DIRECTION('ref_axis',(-0.707106781186548,0.,0.707106781186547));
#14122=DIRECTION('',(0.707106781186548,0.,-0.707106781186547));
#14123=DIRECTION('',(0.707106781186548,0.,-0.707106781186547));
#14124=DIRECTION('center_axis',(0.707106781186547,0.,0.707106781186548));
#14125=DIRECTION('ref_axis',(0.707106781186548,0.,-0.707106781186547));
#14126=DIRECTION('',(0.707106781186548,0.,-0.707106781186547));
#14127=DIRECTION('',(-0.707106781186548,0.,0.707106781186547));
#14128=DIRECTION('center_axis',(-0.707106781186546,0.,-0.707106781186549));
#14129=DIRECTION('ref_axis',(-0.707106781186549,0.,0.707106781186546));
#14130=DIRECTION('',(0.707106781186549,0.,-0.707106781186546));
#14131=DIRECTION('',(0.,1.,0.));
#14132=DIRECTION('',(0.707106781186549,0.,-0.707106781186546));
#14133=DIRECTION('',(0.,1.,0.));
#14134=DIRECTION('center_axis',(-1.,0.,-9.63657966750171E-16));
#14135=DIRECTION('ref_axis',(-9.63657966750171E-16,0.,1.));
#14136=DIRECTION('',(-9.63657966750171E-16,0.,1.));
#14137=DIRECTION('',(0.,1.,0.));
#14138=DIRECTION('',(9.63657966750171E-16,0.,-1.));
#14139=DIRECTION('center_axis',(-9.63657966750171E-16,0.,1.));
#14140=DIRECTION('ref_axis',(1.,0.,9.63657966750171E-16));
#14141=DIRECTION('',(1.,0.,9.63657966750171E-16));
#14142=DIRECTION('',(-1.,0.,-9.63657966750171E-16));
#14143=DIRECTION('center_axis',(-1.02489030670754E-15,0.,1.));
#14144=DIRECTION('ref_axis',(1.,0.,1.02489030670754E-15));
#14145=DIRECTION('',(-1.,0.,-1.02489030670754E-15));
#14146=DIRECTION('',(0.,1.,0.));
#14147=DIRECTION('',(-1.,0.,-1.02489030670754E-15));
#14148=DIRECTION('',(0.,1.,0.));
#14149=DIRECTION('center_axis',(-0.707106781186548,0.,0.707106781186547));
#14150=DIRECTION('ref_axis',(0.707106781186547,0.,0.707106781186548));
#14151=DIRECTION('',(-0.707106781186547,0.,-0.707106781186548));
#14152=DIRECTION('',(-0.707106781186547,0.,-0.707106781186548));
#14153=DIRECTION('center_axis',(0.707106781186548,0.,-0.707106781186547));
#14154=DIRECTION('ref_axis',(-0.707106781186547,0.,-0.707106781186548));
#14155=DIRECTION('',(-0.707106781186547,0.,-0.707106781186548));
#14156=DIRECTION('',(0.,1.,0.));
#14157=DIRECTION('',(0.707106781186547,0.,0.707106781186548));
#14158=DIRECTION('center_axis',(1.,0.,-3.41138552080488E-16));
#14159=DIRECTION('ref_axis',(-3.41138552080488E-16,0.,-1.));
#14160=DIRECTION('',(-3.41138552080488E-16,0.,-1.));
#14161=DIRECTION('',(0.,1.,0.));
#14162=DIRECTION('',(3.41138552080488E-16,0.,1.));
#14163=DIRECTION('center_axis',(-1.03278883703701E-16,0.,1.));
#14164=DIRECTION('ref_axis',(1.,0.,1.03278883703701E-16));
#14165=DIRECTION('',(-1.,0.,-1.03278883703701E-16));
#14166=DIRECTION('',(0.,1.,0.));
#14167=DIRECTION('',(-1.,0.,-1.03278883703701E-16));
#14168=DIRECTION('center_axis',(1.,0.,1.02489030670754E-15));
#14169=DIRECTION('ref_axis',(1.02489030670754E-15,0.,-1.));
#14170=DIRECTION('',(-1.02489030670754E-15,0.,1.));
#14171=DIRECTION('',(0.,1.,0.));
#14172=DIRECTION('',(-1.02489030670754E-15,0.,1.));
#14173=DIRECTION('center_axis',(0.707106781186548,0.,-0.707106781186547));
#14174=DIRECTION('ref_axis',(-0.707106781186547,0.,-0.707106781186548));
#14175=DIRECTION('',(-0.707106781186547,0.,-0.707106781186548));
#14176=DIRECTION('',(0.,1.,0.));
#14177=DIRECTION('',(0.707106781186547,0.,0.707106781186548));
#14178=DIRECTION('center_axis',(5.73677493311137E-16,0.,-1.));
#14179=DIRECTION('ref_axis',(-1.,0.,-5.73677493311137E-16));
#14180=DIRECTION('',(-1.,0.,-5.73677493311137E-16));
#14181=DIRECTION('',(0.,1.,0.));
#14182=DIRECTION('',(1.,0.,5.73677493311137E-16));
#14183=DIRECTION('center_axis',(0.,-1.,0.));
#14184=DIRECTION('ref_axis',(1.,0.,7.68622845445844E-15));
#14185=DIRECTION('center_axis',(0.,-1.,0.));
#14186=DIRECTION('ref_axis',(1.,0.,7.68622845445844E-15));
#14187=DIRECTION('',(0.,1.,0.));
#14188=DIRECTION('center_axis',(0.,1.,0.));
#14189=DIRECTION('ref_axis',(1.,0.,7.68622845445844E-15));
#14190=DIRECTION('center_axis',(-1.,0.,-1.02489030670754E-15));
#14191=DIRECTION('ref_axis',(-1.02489030670754E-15,0.,1.));
#14192=DIRECTION('',(-1.02489030670754E-15,0.,1.));
#14193=DIRECTION('',(0.,1.,0.));
#14194=DIRECTION('',(1.02489030670754E-15,0.,-1.));
#14195=DIRECTION('center_axis',(-0.707106781186549,0.,0.707106781186546));
#14196=DIRECTION('ref_axis',(0.707106781186546,0.,0.707106781186549));
#14197=DIRECTION('',(-0.707106781186546,0.,-0.707106781186549));
#14198=DIRECTION('',(0.,1.,0.));
#14199=DIRECTION('',(-0.707106781186546,0.,-0.707106781186549));
#14200=DIRECTION('center_axis',(-1.02489030670754E-15,0.,1.));
#14201=DIRECTION('ref_axis',(1.,0.,1.02489030670754E-15));
#14202=DIRECTION('',(1.,0.,1.02489030670754E-15));
#14203=DIRECTION('',(0.,1.,0.));
#14204=DIRECTION('',(-1.,0.,-1.02489030670754E-15));
#14205=DIRECTION('center_axis',(1.,0.,1.02489030670754E-15));
#14206=DIRECTION('ref_axis',(1.02489030670754E-15,0.,-1.));
#14207=DIRECTION('',(1.02489030670754E-15,0.,-1.));
#14208=DIRECTION('',(-1.02489030670754E-15,0.,1.));
#14209=DIRECTION('center_axis',(0.707106781186548,0.,-0.707106781186547));
#14210=DIRECTION('ref_axis',(-0.707106781186547,0.,-0.707106781186548));
#14211=DIRECTION('',(0.707106781186547,0.,0.707106781186548));
#14212=DIRECTION('',(0.707106781186547,0.,0.707106781186548));
#14213=DIRECTION('center_axis',(-0.707106781186548,0.,0.707106781186547));
#14214=DIRECTION('ref_axis',(0.707106781186547,0.,0.707106781186548));
#14215=DIRECTION('',(0.707106781186547,0.,0.707106781186548));
#14216=DIRECTION('',(0.,1.,0.));
#14217=DIRECTION('',(-0.707106781186547,0.,-0.707106781186548));
#14218=DIRECTION('center_axis',(-1.,0.,4.63603231995223E-16));
#14219=DIRECTION('ref_axis',(4.63603231995223E-16,0.,1.));
#14220=DIRECTION('',(4.63603231995223E-16,0.,1.));
#14221=DIRECTION('',(0.,1.,0.));
#14222=DIRECTION('',(-4.63603231995223E-16,0.,-1.));
#14223=DIRECTION('center_axis',(-1.91857962110348E-17,0.,-1.));
#14224=DIRECTION('ref_axis',(-1.,0.,1.91857962110348E-17));
#14225=DIRECTION('',(1.,0.,-1.91857962110348E-17));
#14226=DIRECTION('',(0.,1.,0.));
#14227=DIRECTION('',(1.,0.,-1.91857962110348E-17));
#14228=DIRECTION('center_axis',(-1.,0.,-9.02425626792803E-16));
#14229=DIRECTION('ref_axis',(-9.02425626792803E-16,0.,1.));
#14230=DIRECTION('',(9.02425626792803E-16,0.,-1.));
#14231=DIRECTION('',(0.,1.,0.));
#14232=DIRECTION('',(9.02425626792803E-16,0.,-1.));
#14233=DIRECTION('center_axis',(-0.707106781186548,0.,0.707106781186547));
#14234=DIRECTION('ref_axis',(0.707106781186547,0.,0.707106781186548));
#14235=DIRECTION('',(0.707106781186547,0.,0.707106781186548));
#14236=DIRECTION('',(0.,1.,0.));
#14237=DIRECTION('',(-0.707106781186547,0.,-0.707106781186548));
#14238=DIRECTION('center_axis',(4.94455241362763E-16,0.,1.));
#14239=DIRECTION('ref_axis',(1.,0.,-4.94455241362763E-16));
#14240=DIRECTION('',(-1.,0.,4.94455241362763E-16));
#14241=DIRECTION('',(-1.,0.,4.94455241362763E-16));
#14242=DIRECTION('',(0.,1.,0.));
#14243=DIRECTION('center_axis',(1.,0.,0.));
#14244=DIRECTION('ref_axis',(0.,0.,-1.));
#14245=DIRECTION('',(0.,0.,1.));
#14246=DIRECTION('',(0.,0.,1.));
#14247=DIRECTION('',(0.,1.,0.));
#14248=DIRECTION('center_axis',(0.,1.,0.));
#14249=DIRECTION('ref_axis',(-1.,0.,-1.22464679914735E-16));
#14250=DIRECTION('',(1.,0.,4.51212813396402E-16));
#14251=DIRECTION('',(1.,0.,6.12323399573677E-17));
#14252=DIRECTION('',(-0.707106781186548,0.,-0.707106781186547));
#14253=DIRECTION('',(-6.12323399573677E-17,0.,1.));
#14254=DIRECTION('',(-1.,0.,-6.12323399573677E-17));
#14255=DIRECTION('',(6.12323399573677E-17,0.,-1.));
#14256=DIRECTION('',(-0.707106781186547,0.,-0.707106781186548));
#14257=DIRECTION('',(1.,0.,0.));
#14258=DIRECTION('',(0.707106781186548,0.,-0.707106781186547));
#14259=DIRECTION('',(1.36602885878803E-15,0.,-1.));
#14260=DIRECTION('',(1.,0.,9.21611423003838E-16));
#14261=DIRECTION('',(0.,0.,1.));
#14262=DIRECTION('',(0.707106781186548,0.,-0.707106781186547));
#14263=DIRECTION('',(1.,0.,4.51212813396402E-16));
#14264=DIRECTION('center_axis',(0.,1.,0.));
#14265=DIRECTION('ref_axis',(-1.,0.,6.6613381477509E-15));
#14266=DIRECTION('',(0.,0.,1.));
#14267=DIRECTION('',(0.707106781186547,0.,-0.707106781186548));
#14268=DIRECTION('',(-1.,0.,0.));
#14269=DIRECTION('',(0.,0.,-1.));
#14270=DIRECTION('',(1.,0.,0.));
#14271=DIRECTION('',(0.707106781186548,0.,-0.707106781186547));
#14272=DIRECTION('',(0.,0.,1.));
#14273=DIRECTION('',(0.707106781186547,0.,0.707106781186548));
#14274=DIRECTION('',(1.,0.,1.54972587866013E-15));
#14275=DIRECTION('',(-1.10530844287594E-15,0.,1.));
#14276=DIRECTION('',(-1.,0.,-1.83697019872103E-16));
#14277=DIRECTION('',(0.707106781186547,0.,0.707106781186548));
#14278=DIRECTION('',(-6.34909833268504E-16,0.,1.));
#14279=DIRECTION('center_axis',(0.,1.,0.));
#14280=DIRECTION('ref_axis',(-6.4776411278788E-15,0.,-1.));
#14281=DIRECTION('',(-1.,0.,-1.83697019872103E-16));
#14282=DIRECTION('',(0.707106781186548,0.,0.707106781186547));
#14283=DIRECTION('',(1.83697019872103E-16,0.,-1.));
#14284=DIRECTION('',(1.,0.,1.83697019872103E-16));
#14285=DIRECTION('',(-1.83697019872103E-16,0.,1.));
#14286=DIRECTION('',(0.707106781186547,0.,0.707106781186548));
#14287=DIRECTION('',(-1.,0.,0.));
#14288=DIRECTION('',(-0.707106781186548,0.,0.707106781186547));
#14289=DIRECTION('',(-1.48849353870276E-15,0.,1.));
#14290=DIRECTION('',(-1.,0.,-1.04407610291857E-15));
#14291=DIRECTION('',(1.22464679914735E-16,0.,-1.));
#14292=DIRECTION('',(-0.707106781186548,0.,0.707106781186547));
#14293=DIRECTION('',(-0.707106781186548,0.,0.707106781186547));
#14294=DIRECTION('',(0.,0.,-1.));
#14295=DIRECTION('',(-0.707106781186547,0.,-0.707106781186548));
#14296=DIRECTION('',(0.,0.,1.));
#14297=DIRECTION('',(1.,0.,4.94455241362763E-16));
#14298=DIRECTION('center_axis',(0.,-1.,0.));
#14299=DIRECTION('ref_axis',(1.,0.,0.));
#14300=DIRECTION('center_axis',(-4.94455241362763E-16,0.,1.));
#14301=DIRECTION('ref_axis',(1.,0.,4.94455241362763E-16));
#14302=DIRECTION('',(0.,1.,0.));
#14303=DIRECTION('',(1.,0.,4.94455241362763E-16));
#14304=DIRECTION('center_axis',(-1.,0.,0.));
#14305=DIRECTION('ref_axis',(0.,0.,1.));
#14306=DIRECTION('',(0.,1.,0.));
#14307=DIRECTION('',(0.,0.,1.));
#14308=DIRECTION('center_axis',(1.,0.,0.));
#14309=DIRECTION('ref_axis',(0.,0.,-1.));
#14310=DIRECTION('',(0.,1.,0.));
#14311=DIRECTION('',(0.,0.,-1.));
#14312=DIRECTION('',(0.,1.,0.));
#14313=DIRECTION('center_axis',(0.,0.,1.));
#14314=DIRECTION('ref_axis',(1.,0.,0.));
#14315=DIRECTION('',(0.,1.,0.));
#14316=DIRECTION('',(0.,1.,0.));
#14317=DIRECTION('',(1.,0.,0.));
#14318=DIRECTION('center_axis',(-1.,0.,0.));
#14319=DIRECTION('ref_axis',(0.,0.,1.));
#14320=DIRECTION('',(0.,1.,0.));
#14321=DIRECTION('',(0.,0.,1.));
#14322=DIRECTION('',(0.,1.,0.));
#14323=DIRECTION('center_axis',(0.,1.,0.));
#14324=DIRECTION('ref_axis',(1.,0.,0.));
#14325=DIRECTION('',(0.,1.,0.));
#14326=DIRECTION('center_axis',(0.,-1.,0.));
#14327=DIRECTION('ref_axis',(1.,0.,0.));
#14328=DIRECTION('center_axis',(0.,0.,-1.));
#14329=DIRECTION('ref_axis',(-1.,0.,0.));
#14330=DIRECTION('',(0.,1.,0.));
#14331=DIRECTION('',(0.,1.,0.));
#14332=DIRECTION('',(-1.,0.,0.));
#14333=DIRECTION('center_axis',(1.,0.,1.83697019872103E-16));
#14334=DIRECTION('ref_axis',(1.83697019872103E-16,0.,-1.));
#14335=DIRECTION('',(0.,1.,0.));
#14336=DIRECTION('',(1.83697019872103E-16,0.,-1.));
#14337=DIRECTION('',(0.,1.,0.));
#14338=DIRECTION('center_axis',(0.707106781186548,0.,-0.707106781186547));
#14339=DIRECTION('ref_axis',(-0.707106781186547,0.,-0.707106781186548));
#14340=DIRECTION('',(-0.707106781186547,0.,-0.707106781186548));
#14341=DIRECTION('center_axis',(-0.707106781186548,0.,0.707106781186547));
#14342=DIRECTION('ref_axis',(0.707106781186547,0.,0.707106781186548));
#14343=DIRECTION('',(0.707106781186547,0.,0.707106781186548));
#14344=DIRECTION('',(0.,1.,0.));
#14345=DIRECTION('center_axis',(-1.54972587866013E-15,0.,1.));
#14346=DIRECTION('ref_axis',(1.,0.,1.54972587866013E-15));
#14347=DIRECTION('',(1.,0.,1.54972587866013E-15));
#14348=DIRECTION('',(0.,1.,0.));
#14349=DIRECTION('center_axis',(1.,0.,1.10530844287594E-15));
#14350=DIRECTION('ref_axis',(1.10530844287594E-15,0.,-1.));
#14351=DIRECTION('',(1.10530844287594E-15,0.,-1.));
#14352=DIRECTION('',(0.,1.,0.));
#14353=DIRECTION('center_axis',(-1.83697019872103E-16,0.,1.));
#14354=DIRECTION('ref_axis',(1.,0.,1.83697019872103E-16));
#14355=DIRECTION('',(1.,0.,1.83697019872103E-16));
#14356=DIRECTION('',(0.,1.,0.));
#14357=DIRECTION('center_axis',(-0.707106781186548,0.,0.707106781186547));
#14358=DIRECTION('ref_axis',(0.707106781186547,0.,0.707106781186548));
#14359=DIRECTION('',(0.707106781186547,0.,0.707106781186548));
#14360=DIRECTION('',(0.,1.,0.));
#14361=DIRECTION('center_axis',(-1.,0.,-6.34909833268504E-16));
#14362=DIRECTION('ref_axis',(-6.34909833268504E-16,0.,1.));
#14363=DIRECTION('',(-6.34909833268504E-16,0.,1.));
#14364=DIRECTION('',(0.,1.,0.));
#14365=DIRECTION('center_axis',(0.,1.,0.));
#14366=DIRECTION('ref_axis',(-6.4776411278788E-15,0.,-1.));
#14367=DIRECTION('center_axis',(0.,1.,0.));
#14368=DIRECTION('ref_axis',(-6.4776411278788E-15,0.,-1.));
#14369=DIRECTION('',(0.,1.,0.));
#14370=DIRECTION('center_axis',(1.83697019872103E-16,0.,-1.));
#14371=DIRECTION('ref_axis',(-1.,0.,-1.83697019872103E-16));
#14372=DIRECTION('',(-1.,0.,-1.83697019872103E-16));
#14373=DIRECTION('',(0.,1.,0.));
#14374=DIRECTION('center_axis',(0.707106781186547,0.,-0.707106781186548));
#14375=DIRECTION('ref_axis',(-0.707106781186548,0.,-0.707106781186547));
#14376=DIRECTION('',(-0.707106781186548,0.,-0.707106781186547));
#14377=DIRECTION('',(0.,1.,0.));
#14378=DIRECTION('center_axis',(1.,0.,1.83697019872103E-16));
#14379=DIRECTION('ref_axis',(1.83697019872103E-16,0.,-1.));
#14380=DIRECTION('',(1.83697019872103E-16,0.,-1.));
#14381=DIRECTION('',(0.,1.,0.));
#14382=DIRECTION('center_axis',(-1.83697019872103E-16,0.,1.));
#14383=DIRECTION('ref_axis',(1.,0.,1.83697019872103E-16));
#14384=DIRECTION('',(1.,0.,1.83697019872103E-16));
#14385=DIRECTION('center_axis',(-1.,0.,-6.12323399573677E-17));
#14386=DIRECTION('ref_axis',(-6.12323399573677E-17,0.,1.));
#14387=DIRECTION('',(0.,1.,0.));
#14388=DIRECTION('',(-6.12323399573677E-17,0.,1.));
#14389=DIRECTION('',(0.,1.,0.));
#14390=DIRECTION('center_axis',(-0.707106781186548,0.,0.707106781186547));
#14391=DIRECTION('ref_axis',(0.707106781186547,0.,0.707106781186548));
#14392=DIRECTION('',(0.707106781186547,0.,0.707106781186548));
#14393=DIRECTION('center_axis',(0.707106781186548,0.,-0.707106781186547));
#14394=DIRECTION('ref_axis',(-0.707106781186547,0.,-0.707106781186548));
#14395=DIRECTION('',(-0.707106781186547,0.,-0.707106781186548));
#14396=DIRECTION('center_axis',(-6.12323399573677E-17,0.,1.));
#14397=DIRECTION('ref_axis',(1.,0.,6.12323399573677E-17));
#14398=DIRECTION('',(1.,0.,6.12323399573677E-17));
#14399=DIRECTION('',(0.,1.,0.));
#14400=DIRECTION('center_axis',(-0.707106781186547,0.,0.707106781186548));
#14401=DIRECTION('ref_axis',(0.707106781186548,0.,0.707106781186547));
#14402=DIRECTION('',(0.707106781186548,0.,0.707106781186547));
#14403=DIRECTION('',(0.,1.,0.));
#14404=DIRECTION('center_axis',(-1.,0.,-6.12323399573677E-17));
#14405=DIRECTION('ref_axis',(-6.12323399573677E-17,0.,1.));
#14406=DIRECTION('',(-6.12323399573677E-17,0.,1.));
#14407=DIRECTION('',(0.,1.,0.));
#14408=DIRECTION('center_axis',(6.12323399573677E-17,0.,-1.));
#14409=DIRECTION('ref_axis',(-1.,0.,-6.12323399573677E-17));
#14410=DIRECTION('',(-1.,0.,-6.12323399573677E-17));
#14411=DIRECTION('center_axis',(0.,0.,-1.));
#14412=DIRECTION('ref_axis',(-1.,0.,0.));
#14413=DIRECTION('',(0.,1.,0.));
#14414=DIRECTION('',(-1.,0.,0.));
#14415=DIRECTION('',(0.,1.,0.));
#14416=DIRECTION('center_axis',(-0.707106781186547,0.,-0.707106781186548));
#14417=DIRECTION('ref_axis',(-0.707106781186548,0.,0.707106781186547));
#14418=DIRECTION('',(-0.707106781186548,0.,0.707106781186547));
#14419=DIRECTION('center_axis',(0.707106781186547,0.,0.707106781186548));
#14420=DIRECTION('ref_axis',(0.707106781186548,0.,-0.707106781186547));
#14421=DIRECTION('',(0.707106781186548,0.,-0.707106781186547));
#14422=DIRECTION('',(0.,1.,0.));
#14423=DIRECTION('center_axis',(1.,0.,1.36602885878803E-15));
#14424=DIRECTION('ref_axis',(1.36602885878803E-15,0.,-1.));
#14425=DIRECTION('',(1.36602885878803E-15,0.,-1.));
#14426=DIRECTION('',(0.,1.,0.));
#14427=DIRECTION('center_axis',(9.21611423003838E-16,0.,-1.));
#14428=DIRECTION('ref_axis',(-1.,0.,-9.21611423003838E-16));
#14429=DIRECTION('',(-1.,0.,-9.21611423003838E-16));
#14430=DIRECTION('',(0.,1.,0.));
#14431=DIRECTION('center_axis',(1.,0.,0.));
#14432=DIRECTION('ref_axis',(0.,0.,-1.));
#14433=DIRECTION('',(0.,0.,-1.));
#14434=DIRECTION('',(0.,1.,0.));
#14435=DIRECTION('center_axis',(0.707106781186547,0.,0.707106781186548));
#14436=DIRECTION('ref_axis',(0.707106781186548,0.,-0.707106781186547));
#14437=DIRECTION('',(0.707106781186548,0.,-0.707106781186547));
#14438=DIRECTION('',(0.,1.,0.));
#14439=DIRECTION('center_axis',(-4.51212813396402E-16,0.,1.));
#14440=DIRECTION('ref_axis',(1.,0.,4.51212813396402E-16));
#14441=DIRECTION('',(1.,0.,4.51212813396402E-16));
#14442=DIRECTION('',(0.,1.,0.));
#14443=DIRECTION('center_axis',(0.,1.,0.));
#14444=DIRECTION('ref_axis',(-1.,0.,6.6613381477509E-15));
#14445=DIRECTION('center_axis',(0.,1.,0.));
#14446=DIRECTION('ref_axis',(-1.,0.,6.6613381477509E-15));
#14447=DIRECTION('',(0.,1.,0.));
#14448=DIRECTION('center_axis',(-1.,0.,0.));
#14449=DIRECTION('ref_axis',(0.,0.,1.));
#14450=DIRECTION('',(0.,0.,1.));
#14451=DIRECTION('',(0.,1.,0.));
#14452=DIRECTION('center_axis',(-0.707106781186548,0.,-0.707106781186547));
#14453=DIRECTION('ref_axis',(-0.707106781186547,0.,0.707106781186548));
#14454=DIRECTION('',(-0.707106781186547,0.,0.707106781186548));
#14455=DIRECTION('',(0.,1.,0.));
#14456=DIRECTION('center_axis',(0.,0.,-1.));
#14457=DIRECTION('ref_axis',(-1.,0.,0.));
#14458=DIRECTION('',(-1.,0.,0.));
#14459=DIRECTION('',(0.,1.,0.));
#14460=DIRECTION('center_axis',(1.,0.,0.));
#14461=DIRECTION('ref_axis',(0.,0.,-1.));
#14462=DIRECTION('',(0.,0.,-1.));
#14463=DIRECTION('center_axis',(0.707106781186547,0.,0.707106781186548));
#14464=DIRECTION('ref_axis',(0.707106781186548,0.,-0.707106781186547));
#14465=DIRECTION('',(0.707106781186548,0.,-0.707106781186547));
#14466=DIRECTION('center_axis',(-0.707106781186547,0.,-0.707106781186548));
#14467=DIRECTION('ref_axis',(-0.707106781186548,0.,0.707106781186547));
#14468=DIRECTION('',(-0.707106781186548,0.,0.707106781186547));
#14469=DIRECTION('',(0.,1.,0.));
#14470=DIRECTION('center_axis',(-1.,0.,-1.48849353870276E-15));
#14471=DIRECTION('ref_axis',(-1.48849353870276E-15,0.,1.));
#14472=DIRECTION('',(-1.48849353870276E-15,0.,1.));
#14473=DIRECTION('',(0.,1.,0.));
#14474=DIRECTION('center_axis',(-1.04407610291857E-15,0.,1.));
#14475=DIRECTION('ref_axis',(1.,0.,1.04407610291857E-15));
#14476=DIRECTION('',(1.,0.,1.04407610291857E-15));
#14477=DIRECTION('',(0.,1.,0.));
#14478=DIRECTION('center_axis',(-1.,0.,-1.22464679914735E-16));
#14479=DIRECTION('ref_axis',(-1.22464679914735E-16,0.,1.));
#14480=DIRECTION('',(-1.22464679914735E-16,0.,1.));
#14481=DIRECTION('',(0.,1.,0.));
#14482=DIRECTION('center_axis',(-0.707106781186547,0.,-0.707106781186548));
#14483=DIRECTION('ref_axis',(-0.707106781186548,0.,0.707106781186547));
#14484=DIRECTION('',(-0.707106781186548,0.,0.707106781186547));
#14485=DIRECTION('',(0.,1.,0.));
#14486=DIRECTION('center_axis',(5.73677493311137E-16,0.,-1.));
#14487=DIRECTION('ref_axis',(-1.,0.,-5.73677493311137E-16));
#14488=DIRECTION('',(-1.,0.,-5.73677493311137E-16));
#14489=DIRECTION('center_axis',(0.,1.,0.));
#14490=DIRECTION('ref_axis',(-1.,0.,-1.22464679914735E-16));
#34884=CARTESIAN_POINT('',(0.,0.,0.));
#34885=CARTESIAN_POINT('Origin',(2.69069170170099,0.,-6.2440918089009));
#34886=CARTESIAN_POINT('',(2.69069170170099,0.,-8.19999999999999));
#34887=CARTESIAN_POINT('',(2.69069170170099,0.,-6.2440918089009));
#34888=CARTESIAN_POINT('',(2.69069170170099,0.,-6.33074178210092));
#34889=CARTESIAN_POINT('',(2.69069170170099,500.,-6.2440918089009));
#34890=CARTESIAN_POINT('',(2.69069170170099,0.,-6.2440918089009));
#34891=CARTESIAN_POINT('',(2.69069170170099,500.,-8.19999999999999));
#34892=CARTESIAN_POINT('',(2.69069170170099,500.,-6.33074178210092));
#34893=CARTESIAN_POINT('',(2.69069170170099,0.,-8.19999999999999));
#34894=CARTESIAN_POINT('Origin',(2.69069170170097,0.,6.24409180890091));
#34895=CARTESIAN_POINT('',(2.69069170170097,0.,6.24409180890091));
#34896=CARTESIAN_POINT('',(2.69069170170097,0.,8.2));
#34897=CARTESIAN_POINT('',(2.69069170170098,0.,-0.0866499732000153));
#34898=CARTESIAN_POINT('',(2.69069170170097,500.,8.2));
#34899=CARTESIAN_POINT('',(2.69069170170097,0.,8.2));
#34900=CARTESIAN_POINT('',(2.69069170170097,500.,6.24409180890091));
#34901=CARTESIAN_POINT('',(2.69069170170098,500.,-0.0866499732000138));
#34902=CARTESIAN_POINT('',(2.69069170170097,0.,6.24409180890091));
#34903=CARTESIAN_POINT('Origin',(6.09999999999999,0.,3.90000000000001));
#34904=CARTESIAN_POINT('',(6.1,0.,-2.83478351060188));
#34905=CARTESIAN_POINT('',(6.1,500.,-2.83478351060188));
#34906=CARTESIAN_POINT('',(6.1,0.,-2.83478351060188));
#34907=CARTESIAN_POINT('',(6.09999999999999,0.,2.8347835106019));
#34908=CARTESIAN_POINT('',(6.09999999999999,0.,3.90000000000001));
#34909=CARTESIAN_POINT('',(6.09999999999999,500.,2.8347835106019));
#34910=CARTESIAN_POINT('',(6.09999999999999,0.,2.8347835106019));
#34911=CARTESIAN_POINT('',(6.1,500.,-1.25869587765046));
#34912=CARTESIAN_POINT('Origin',(13.9,0.,3.90000000000001));
#34913=CARTESIAN_POINT('',(12.8347835106019,0.,3.90000000000001));
#34914=CARTESIAN_POINT('',(12.8347835106019,500.,3.90000000000001));
#34915=CARTESIAN_POINT('',(12.8347835106019,0.,3.90000000000001));
#34916=CARTESIAN_POINT('',(7.1652164893981,500.,3.90000000000001));
#34917=CARTESIAN_POINT('',(5.15869587765046,500.,3.90000000000001));
#34918=CARTESIAN_POINT('',(7.1652164893981,0.,3.90000000000001));
#34919=CARTESIAN_POINT('',(7.1652164893981,0.,3.90000000000001));
#34920=CARTESIAN_POINT('',(13.9,0.,3.90000000000001));
#34921=CARTESIAN_POINT('Origin',(13.9,0.,-3.89999999999999));
#34922=CARTESIAN_POINT('',(13.9,0.,2.8347835106019));
#34923=CARTESIAN_POINT('',(13.9,500.,2.8347835106019));
#34924=CARTESIAN_POINT('',(13.9,0.,2.8347835106019));
#34925=CARTESIAN_POINT('',(13.9,0.,-2.83478351060188));
#34926=CARTESIAN_POINT('',(13.9,0.,-3.89999999999999));
#34927=CARTESIAN_POINT('',(13.9,500.,-2.83478351060188));
#34928=CARTESIAN_POINT('',(13.9,0.,-2.83478351060188));
#34929=CARTESIAN_POINT('',(13.9,500.,-5.15869587765045));
#34930=CARTESIAN_POINT('Origin',(10.,0.,1.02489030670754E-14));
#34931=CARTESIAN_POINT('',(12.1,500.,1.26583485389822E-14));
#34932=CARTESIAN_POINT('Origin',(10.,500.,1.02489030670754E-14));
#34933=CARTESIAN_POINT('',(12.1,0.,1.26583485389822E-14));
#34934=CARTESIAN_POINT('',(12.1,0.,1.26583485389822E-14));
#34935=CARTESIAN_POINT('Origin',(10.,0.,1.02489030670754E-14));
#34936=CARTESIAN_POINT('Origin',(6.1,0.,-3.89999999999999));
#34937=CARTESIAN_POINT('',(7.16521648939811,0.,-3.89999999999999));
#34938=CARTESIAN_POINT('',(7.16521648939811,500.,-3.89999999999999));
#34939=CARTESIAN_POINT('',(7.16521648939811,0.,-3.89999999999999));
#34940=CARTESIAN_POINT('',(12.8347835106019,500.,-3.89999999999999));
#34941=CARTESIAN_POINT('',(1.25869587765047,500.,-3.9));
#34942=CARTESIAN_POINT('',(12.8347835106019,0.,-3.89999999999999));
#34943=CARTESIAN_POINT('',(12.8347835106019,0.,-3.89999999999999));
#34944=CARTESIAN_POINT('',(6.1,0.,-3.89999999999999));
#34945=CARTESIAN_POINT('Origin',(15.509308298299,0.,-6.57452478769711));
#34946=CARTESIAN_POINT('',(15.509308298299,0.,-8.19999999999998));
#34947=CARTESIAN_POINT('',(15.509308298299,0.,-6.57452478769711));
#34948=CARTESIAN_POINT('',(15.509308298299,0.,-8.19999999999998));
#34949=CARTESIAN_POINT('',(15.509308298299,500.,-6.57452478769711));
#34950=CARTESIAN_POINT('',(15.509308298299,0.,-6.57452478769711));
#34951=CARTESIAN_POINT('',(15.509308298299,500.,-8.19999999999998));
#34952=CARTESIAN_POINT('',(15.509308298299,500.,-6.49595827149902));
#34953=CARTESIAN_POINT('',(15.509308298299,0.,-8.19999999999998));
#34954=CARTESIAN_POINT('Origin',(12.8347835106019,0.,-3.89999999999999));
#34955=CARTESIAN_POINT('',(15.509308298299,0.,-6.57452478769711));
#34956=CARTESIAN_POINT('',(9.35978351060189,500.,-0.424999999999988));
#34957=CARTESIAN_POINT('Origin',(16.5745247876971,0.,-5.509308298299));
#34958=CARTESIAN_POINT('',(16.5745247876971,0.,-5.509308298299));
#34959=CARTESIAN_POINT('',(16.5745247876971,0.,-5.509308298299));
#34960=CARTESIAN_POINT('',(16.5745247876971,500.,-5.509308298299));
#34961=CARTESIAN_POINT('',(16.5745247876971,0.,-5.509308298299));
#34962=CARTESIAN_POINT('',(11.7622623938486,500.,-0.697045904450441));
#34963=CARTESIAN_POINT('Origin',(18.2,0.,-5.509308298299));
#34964=CARTESIAN_POINT('',(18.2,0.,-5.509308298299));
#34965=CARTESIAN_POINT('',(18.2,0.,-5.509308298299));
#34966=CARTESIAN_POINT('',(18.2,500.,-5.509308298299));
#34967=CARTESIAN_POINT('',(18.2,0.,-5.509308298299));
#34968=CARTESIAN_POINT('',(7.30869587765047,500.,-5.509308298299));
#34969=CARTESIAN_POINT('Origin',(18.2,0.,-3.09999999999998));
#34970=CARTESIAN_POINT('',(18.2,0.,-3.09999999999998));
#34971=CARTESIAN_POINT('',(18.2,0.,-5.509308298299));
#34972=CARTESIAN_POINT('',(18.2,500.,-3.09999999999998));
#34973=CARTESIAN_POINT('',(18.2,0.,-3.09999999999998));
#34974=CARTESIAN_POINT('',(18.2,500.,-4.75869587765046));
#34975=CARTESIAN_POINT('Origin',(18.5210615995951,0.,-3.09999999999998));
#34976=CARTESIAN_POINT('',(18.5210615995951,0.,-3.09999999999998));
#34977=CARTESIAN_POINT('',(18.2,0.,-3.09999999999998));
#34978=CARTESIAN_POINT('',(18.5210615995951,500.,-3.09999999999998));
#34979=CARTESIAN_POINT('',(18.5210615995951,0.,-3.09999999999998));
#34980=CARTESIAN_POINT('',(7.46922667744803,500.,-3.09999999999999));
#34981=CARTESIAN_POINT('Origin',(20.,0.,-4.57893840040485));
#34982=CARTESIAN_POINT('',(20.,0.,-4.57893840040485));
#34983=CARTESIAN_POINT('',(20.,0.,-4.57893840040485));
#34984=CARTESIAN_POINT('',(20.,500.,-4.57893840040485));
#34985=CARTESIAN_POINT('',(20.,0.,-4.57893840040485));
#34986=CARTESIAN_POINT('',(14.5639612775493,500.,0.857100322045891));
#34987=CARTESIAN_POINT('Origin',(20.,0.,-9.49999999999998));
#34988=CARTESIAN_POINT('',(20.,0.,-9.49999999999998));
#34989=CARTESIAN_POINT('',(20.,0.,-9.49999999999998));
#34990=CARTESIAN_POINT('',(20.,500.,-9.49999999999998));
#34991=CARTESIAN_POINT('',(20.,0.,-9.49999999999998));
#34992=CARTESIAN_POINT('',(20.,500.,-7.95869587765045));
#34993=CARTESIAN_POINT('Origin',(19.5,0.,-9.49999999999998));
#34994=CARTESIAN_POINT('',(19.5,0.,-9.99999999999998));
#34995=CARTESIAN_POINT('Origin',(19.5,0.,-9.49999999999998));
#34996=CARTESIAN_POINT('',(19.5,500.,-9.99999999999998));
#34997=CARTESIAN_POINT('',(19.5,0.,-9.99999999999998));
#34998=CARTESIAN_POINT('Origin',(19.5,500.,-9.49999999999998));
#34999=CARTESIAN_POINT('Origin',(14.5789384004049,0.,-9.99999999999998));
#35000=CARTESIAN_POINT('',(14.5789384004049,0.,-9.99999999999998));
#35001=CARTESIAN_POINT('',(14.5789384004049,0.,-9.99999999999998));
#35002=CARTESIAN_POINT('',(14.5789384004049,500.,-9.99999999999998));
#35003=CARTESIAN_POINT('',(14.5789384004049,0.,-9.99999999999998));
#35004=CARTESIAN_POINT('',(5.49816507785291,500.,-9.99999999999999));
#35005=CARTESIAN_POINT('Origin',(13.1,0.,-8.52106159959512));
#35006=CARTESIAN_POINT('',(13.1,0.,-8.52106159959512));
#35007=CARTESIAN_POINT('',(14.5789384004049,0.,-9.99999999999998));
#35008=CARTESIAN_POINT('',(13.1,500.,-8.52106159959512));
#35009=CARTESIAN_POINT('',(13.1,0.,-8.52106159959512));
#35010=CARTESIAN_POINT('',(8.40343047775168,500.,-3.82449207734681));
#35011=CARTESIAN_POINT('Origin',(13.1,0.,-8.19999999999998));
#35012=CARTESIAN_POINT('',(13.1,0.,-8.19999999999998));
#35013=CARTESIAN_POINT('',(13.1,0.,-8.19999999999998));
#35014=CARTESIAN_POINT('',(13.1,500.,-8.19999999999998));
#35015=CARTESIAN_POINT('',(13.1,0.,-8.19999999999998));
#35016=CARTESIAN_POINT('',(13.1,500.,-7.30869587765046));
#35017=CARTESIAN_POINT('Origin',(15.509308298299,0.,-8.19999999999998));
#35018=CARTESIAN_POINT('',(15.509308298299,0.,-8.19999999999998));
#35019=CARTESIAN_POINT('',(5.96335002679998,500.,-8.19999999999999));
#35020=CARTESIAN_POINT('Origin',(4.49069170170097,0.,6.57452478769713));
#35021=CARTESIAN_POINT('',(4.49069170170097,0.,8.2));
#35022=CARTESIAN_POINT('',(4.49069170170097,0.,6.57452478769713));
#35023=CARTESIAN_POINT('',(4.49069170170097,0.,8.2));
#35024=CARTESIAN_POINT('',(4.49069170170097,500.,6.57452478769713));
#35025=CARTESIAN_POINT('',(4.49069170170097,0.,6.57452478769713));
#35026=CARTESIAN_POINT('',(4.49069170170097,500.,8.2));
#35027=CARTESIAN_POINT('',(4.49069170170098,500.,0.0785665161980986));
#35028=CARTESIAN_POINT('',(4.49069170170097,0.,8.2));
#35029=CARTESIAN_POINT('Origin',(7.1652164893981,0.,3.90000000000001));
#35030=CARTESIAN_POINT('',(4.49069170170097,0.,6.57452478769713));
#35031=CARTESIAN_POINT('',(7.05760824469904,500.,4.00760824469907));
#35032=CARTESIAN_POINT('Origin',(3.42547521230287,0.,5.50930829829902));
#35033=CARTESIAN_POINT('',(3.42547521230287,0.,5.50930829829902));
#35034=CARTESIAN_POINT('',(4.65512936145237,500.,4.27965414914951));
#35035=CARTESIAN_POINT('Origin',(6.89999999999999,0.,8.52106159959514));
#35036=CARTESIAN_POINT('',(5.42106159959512,0.,10.));
#35037=CARTESIAN_POINT('',(6.89999999999999,0.,8.52106159959514));
#35038=CARTESIAN_POINT('',(5.42106159959512,0.,10.));
#35039=CARTESIAN_POINT('',(6.89999999999999,500.,8.52106159959514));
#35040=CARTESIAN_POINT('',(6.89999999999999,0.,8.52106159959514));
#35041=CARTESIAN_POINT('',(5.42106159959512,500.,10.));
#35042=CARTESIAN_POINT('',(8.01396127754924,500.,7.40710032204589));
#35043=CARTESIAN_POINT('',(5.42106159959512,0.,10.));
#35044=CARTESIAN_POINT('Origin',(6.89999999999999,0.,8.2));
#35045=CARTESIAN_POINT('',(6.89999999999999,0.,8.2));
#35046=CARTESIAN_POINT('',(6.89999999999999,0.,8.2));
#35047=CARTESIAN_POINT('',(6.89999999999999,500.,8.2));
#35048=CARTESIAN_POINT('',(6.89999999999999,0.,8.2));
#35049=CARTESIAN_POINT('',(6.9,500.,0.891304122349535));
#35050=CARTESIAN_POINT('Origin',(4.49069170170097,0.,8.2));
#35051=CARTESIAN_POINT('',(4.49069170170097,0.,8.2));
#35052=CARTESIAN_POINT('',(0.454041728500951,500.,8.2));
#35053=CARTESIAN_POINT('Origin',(16.5745247876971,0.,5.50930829829903));
#35054=CARTESIAN_POINT('',(18.2,0.,5.50930829829903));
#35055=CARTESIAN_POINT('',(16.5745247876971,0.,5.50930829829903));
#35056=CARTESIAN_POINT('',(18.2,0.,5.50930829829903));
#35057=CARTESIAN_POINT('',(16.5745247876971,500.,5.50930829829903));
#35058=CARTESIAN_POINT('',(16.5745247876971,0.,5.50930829829903));
#35059=CARTESIAN_POINT('',(18.2,500.,5.50930829829903));
#35060=CARTESIAN_POINT('',(6.49595827149902,500.,5.50930829829902));
#35061=CARTESIAN_POINT('',(18.2,0.,5.50930829829903));
#35062=CARTESIAN_POINT('Origin',(13.9,0.,2.8347835106019));
#35063=CARTESIAN_POINT('',(16.5745247876971,0.,5.50930829829903));
#35064=CARTESIAN_POINT('',(7.21630412234953,500.,-3.84891236704857));
#35065=CARTESIAN_POINT('Origin',(15.509308298299,0.,6.57452478769714));
#35066=CARTESIAN_POINT('',(15.509308298299,0.,6.57452478769714));
#35067=CARTESIAN_POINT('',(15.509308298299,0.,6.57452478769714));
#35068=CARTESIAN_POINT('',(15.509308298299,500.,6.57452478769714));
#35069=CARTESIAN_POINT('',(15.509308298299,0.,6.57452478769714));
#35070=CARTESIAN_POINT('',(7.48835002679998,500.,-1.4464334838019));
#35071=CARTESIAN_POINT('Origin',(15.509308298299,0.,8.20000000000001));
#35072=CARTESIAN_POINT('',(15.509308298299,0.,8.20000000000001));
#35073=CARTESIAN_POINT('',(15.509308298299,0.,8.20000000000001));
#35074=CARTESIAN_POINT('',(15.509308298299,500.,8.20000000000001));
#35075=CARTESIAN_POINT('',(15.509308298299,0.,8.20000000000001));
#35076=CARTESIAN_POINT('',(15.509308298299,500.,0.891304122349531));
#35077=CARTESIAN_POINT('Origin',(13.1,0.,8.20000000000001));
#35078=CARTESIAN_POINT('',(13.1,0.,8.20000000000001));
#35079=CARTESIAN_POINT('',(15.509308298299,0.,8.20000000000001));
#35080=CARTESIAN_POINT('',(13.1,500.,8.20000000000001));
#35081=CARTESIAN_POINT('',(13.1,0.,8.20000000000001));
#35082=CARTESIAN_POINT('',(4.75869587765046,500.,8.20000000000001));
#35083=CARTESIAN_POINT('Origin',(13.1,0.,8.52106159959514));
#35084=CARTESIAN_POINT('',(13.1,0.,8.52106159959514));
#35085=CARTESIAN_POINT('',(13.1,0.,8.20000000000001));
#35086=CARTESIAN_POINT('',(13.1,500.,8.52106159959514));
#35087=CARTESIAN_POINT('',(13.1,0.,8.52106159959514));
#35088=CARTESIAN_POINT('',(13.1,500.,1.05183492214711));
#35089=CARTESIAN_POINT('Origin',(14.5789384004049,0.,10.));
#35090=CARTESIAN_POINT('',(14.5789384004049,0.,10.));
#35091=CARTESIAN_POINT('',(14.5789384004049,0.,10.));
#35092=CARTESIAN_POINT('',(14.5789384004049,500.,10.));
#35093=CARTESIAN_POINT('',(14.5789384004049,0.,10.));
#35094=CARTESIAN_POINT('',(5.93420380030364,500.,1.35526539989879));
#35095=CARTESIAN_POINT('Origin',(19.5,0.,10.));
#35096=CARTESIAN_POINT('',(19.5,0.,10.));
#35097=CARTESIAN_POINT('',(19.5,0.,10.));
#35098=CARTESIAN_POINT('',(19.5,500.,10.));
#35099=CARTESIAN_POINT('',(19.5,0.,10.));
#35100=CARTESIAN_POINT('',(7.95869587765046,500.,10.));
#35101=CARTESIAN_POINT('Origin',(19.5,0.,9.50000000000001));
#35102=CARTESIAN_POINT('',(20.,0.,9.50000000000001));
#35103=CARTESIAN_POINT('Origin',(19.5,0.,9.50000000000001));
#35104=CARTESIAN_POINT('',(20.,500.,9.50000000000001));
#35105=CARTESIAN_POINT('',(20.,0.,9.50000000000001));
#35106=CARTESIAN_POINT('Origin',(19.5,500.,9.50000000000001));
#35107=CARTESIAN_POINT('Origin',(20.,0.,4.57893840040489));
#35108=CARTESIAN_POINT('',(20.,0.,4.57893840040489));
#35109=CARTESIAN_POINT('',(20.,0.,4.57893840040489));
#35110=CARTESIAN_POINT('',(20.,500.,4.57893840040489));
#35111=CARTESIAN_POINT('',(20.,0.,4.57893840040489));
#35112=CARTESIAN_POINT('',(20.,500.,-0.919226677448016));
#35113=CARTESIAN_POINT('Origin',(18.5210615995951,0.,3.10000000000002));
#35114=CARTESIAN_POINT('',(18.5210615995951,0.,3.10000000000002));
#35115=CARTESIAN_POINT('',(20.,0.,4.57893840040489));
#35116=CARTESIAN_POINT('',(18.5210615995951,500.,3.10000000000002));
#35117=CARTESIAN_POINT('',(18.5210615995951,0.,3.10000000000002));
#35118=CARTESIAN_POINT('',(10.6157961996964,500.,-4.80526539989878));
#35119=CARTESIAN_POINT('Origin',(18.2,0.,3.10000000000002));
#35120=CARTESIAN_POINT('',(18.2,0.,3.10000000000002));
#35121=CARTESIAN_POINT('',(18.2,0.,3.10000000000002));
#35122=CARTESIAN_POINT('',(18.2,500.,3.10000000000002));
#35123=CARTESIAN_POINT('',(18.2,0.,3.10000000000002));
#35124=CARTESIAN_POINT('',(7.30869587765046,500.,3.10000000000001));
#35125=CARTESIAN_POINT('Origin',(18.2,0.,5.50930829829903));
#35126=CARTESIAN_POINT('',(18.2,0.,5.50930829829903));
#35127=CARTESIAN_POINT('',(18.2,500.,-0.454041728500943));
#35128=CARTESIAN_POINT('Origin',(6.1,0.,-2.83478351060188));
#35129=CARTESIAN_POINT('',(3.42547521230287,0.,-5.50930829829901));
#35130=CARTESIAN_POINT('',(2.78369587765047,500.,-6.15108763295141));
#35131=CARTESIAN_POINT('Origin',(4.49069170170099,0.,-6.57452478769712));
#35132=CARTESIAN_POINT('',(4.49069170170099,0.,-6.57452478769712));
#35133=CARTESIAN_POINT('',(4.49069170170099,0.,-6.57452478769712));
#35134=CARTESIAN_POINT('',(4.49069170170099,500.,-6.57452478769712));
#35135=CARTESIAN_POINT('',(4.49069170170099,0.,-6.57452478769712));
#35136=CARTESIAN_POINT('',(2.51164997320002,500.,-8.55356651619809));
#35137=CARTESIAN_POINT('Origin',(4.49069170170099,0.,-8.19999999999999));
#35138=CARTESIAN_POINT('',(4.49069170170099,0.,-8.19999999999999));
#35139=CARTESIAN_POINT('',(4.49069170170099,0.,-8.19999999999999));
#35140=CARTESIAN_POINT('',(4.49069170170099,500.,-8.19999999999999));
#35141=CARTESIAN_POINT('',(4.49069170170099,0.,-8.19999999999999));
#35142=CARTESIAN_POINT('',(4.49069170170099,500.,-7.30869587765047));
#35143=CARTESIAN_POINT('Origin',(6.9,0.,-8.19999999999999));
#35144=CARTESIAN_POINT('',(6.9,0.,-8.19999999999999));
#35145=CARTESIAN_POINT('',(4.49069170170099,0.,-8.19999999999999));
#35146=CARTESIAN_POINT('',(6.9,500.,-8.19999999999999));
#35147=CARTESIAN_POINT('',(6.9,0.,-8.19999999999999));
#35148=CARTESIAN_POINT('',(1.65869587765047,500.,-8.19999999999999));
#35149=CARTESIAN_POINT('Origin',(6.9,0.,-8.52106159959512));
#35150=CARTESIAN_POINT('',(6.9,0.,-8.52106159959512));
#35151=CARTESIAN_POINT('',(6.9,0.,-8.19999999999999));
#35152=CARTESIAN_POINT('',(6.9,500.,-8.52106159959512));
#35153=CARTESIAN_POINT('',(6.9,0.,-8.52106159959512));
#35154=CARTESIAN_POINT('',(6.9,500.,-7.46922667744803));
#35155=CARTESIAN_POINT('Origin',(5.42106159959514,0.,-9.99999999999999));
#35156=CARTESIAN_POINT('',(5.42106159959514,0.,-9.99999999999999));
#35157=CARTESIAN_POINT('',(5.42106159959514,0.,-9.99999999999999));
#35158=CARTESIAN_POINT('',(5.42106159959514,500.,-9.99999999999999));
#35159=CARTESIAN_POINT('',(5.42106159959514,0.,-9.99999999999999));
#35160=CARTESIAN_POINT('',(4.06579619969635,500.,-11.3552653998988));
#35161=CARTESIAN_POINT('Origin',(-2.69069170170098,0.,-8.2));
#35162=CARTESIAN_POINT('',(-2.69069170170098,0.,-8.2));
#35163=CARTESIAN_POINT('',(-3.13664997320002,0.,-8.2));
#35164=CARTESIAN_POINT('',(-2.69069170170098,500.,-8.2));
#35165=CARTESIAN_POINT('',(-3.13664997320002,500.,-8.2));
#35166=CARTESIAN_POINT('',(-2.69069170170098,0.,-8.2));
#35167=CARTESIAN_POINT('Origin',(-2.69069170170098,0.,-6.24409180890091));
#35168=CARTESIAN_POINT('',(-2.69069170170098,0.,-6.24409180890091));
#35169=CARTESIAN_POINT('',(-2.69069170170098,0.,-6.33074178210092));
#35170=CARTESIAN_POINT('',(-2.69069170170098,500.,-6.24409180890091));
#35171=CARTESIAN_POINT('',(-2.69069170170098,500.,-6.33074178210092));
#35172=CARTESIAN_POINT('',(-2.69069170170098,0.,-6.24409180890091));
#35173=CARTESIAN_POINT('Origin',(-3.58260824469906,0.,-6.41739175530094));
#35174=CARTESIAN_POINT('',(-5.42106159959513,0.,-9.99999999999999));
#35175=CARTESIAN_POINT('',(0.500000000000009,0.,-9.99999999999999));
#35176=CARTESIAN_POINT('',(-5.42106159959513,0.,10.));
#35177=CARTESIAN_POINT('',(-5.42106159959513,0.,10.));
#35178=CARTESIAN_POINT('',(-6.9,0.,8.52106159959513));
#35179=CARTESIAN_POINT('',(-5.42106159959513,0.,10.));
#35180=CARTESIAN_POINT('',(-6.9,0.,8.2));
#35181=CARTESIAN_POINT('',(-6.9,0.,8.2));
#35182=CARTESIAN_POINT('',(-4.49069170170099,0.,8.2));
#35183=CARTESIAN_POINT('',(-4.49069170170099,0.,8.2));
#35184=CARTESIAN_POINT('',(-4.49069170170099,0.,6.57452478769713));
#35185=CARTESIAN_POINT('',(-4.49069170170099,0.,8.2));
#35186=CARTESIAN_POINT('',(-7.16521648939811,0.,3.9));
#35187=CARTESIAN_POINT('',(-4.49069170170099,0.,6.57452478769713));
#35188=CARTESIAN_POINT('',(-12.8347835106019,0.,3.9));
#35189=CARTESIAN_POINT('',(-13.9,0.,3.9));
#35190=CARTESIAN_POINT('',(-15.509308298299,0.,6.57452478769712));
#35191=CARTESIAN_POINT('',(-15.509308298299,0.,6.57452478769712));
#35192=CARTESIAN_POINT('',(-15.509308298299,0.,8.19999999999999));
#35193=CARTESIAN_POINT('',(-15.509308298299,0.,8.19999999999999));
#35194=CARTESIAN_POINT('',(-13.1,0.,8.2));
#35195=CARTESIAN_POINT('',(-15.509308298299,0.,8.19999999999999));
#35196=CARTESIAN_POINT('',(-13.1,0.,8.52106159959513));
#35197=CARTESIAN_POINT('',(-13.1,0.,8.2));
#35198=CARTESIAN_POINT('',(-14.5789384004049,0.,10.));
#35199=CARTESIAN_POINT('',(-14.5789384004049,0.,10.));
#35200=CARTESIAN_POINT('',(-19.5,0.,9.99999999999999));
#35201=CARTESIAN_POINT('',(-19.5,0.,9.99999999999999));
#35202=CARTESIAN_POINT('',(-20.,0.,9.49999999999999));
#35203=CARTESIAN_POINT('Origin',(-19.5,0.,9.49999999999999));
#35204=CARTESIAN_POINT('',(-20.,0.,4.57893840040487));
#35205=CARTESIAN_POINT('',(-20.,0.,4.57893840040487));
#35206=CARTESIAN_POINT('',(-18.5210615995951,0.,3.1));
#35207=CARTESIAN_POINT('',(-20.,0.,4.57893840040487));
#35208=CARTESIAN_POINT('',(-18.2,0.,3.1));
#35209=CARTESIAN_POINT('',(-18.2,0.,3.1));
#35210=CARTESIAN_POINT('',(-18.2,0.,5.50930829829901));
#35211=CARTESIAN_POINT('',(-18.2,0.,5.50930829829901));
#35212=CARTESIAN_POINT('',(-16.5745247876971,0.,5.50930829829901));
#35213=CARTESIAN_POINT('',(-18.2,0.,5.50930829829901));
#35214=CARTESIAN_POINT('',(-13.9,0.,2.83478351060189));
#35215=CARTESIAN_POINT('',(-16.5745247876971,0.,5.50930829829901));
#35216=CARTESIAN_POINT('',(-13.9,0.,-2.83478351060189));
#35217=CARTESIAN_POINT('',(-13.9,0.,-3.9));
#35218=CARTESIAN_POINT('',(-16.5745247876971,0.,-5.50930829829902));
#35219=CARTESIAN_POINT('',(-16.5745247876971,0.,-5.50930829829902));
#35220=CARTESIAN_POINT('',(-18.2,0.,-5.50930829829902));
#35221=CARTESIAN_POINT('',(-18.2,0.,-5.50930829829902));
#35222=CARTESIAN_POINT('',(-18.2,0.,-3.1));
#35223=CARTESIAN_POINT('',(-18.2,0.,-5.50930829829902));
#35224=CARTESIAN_POINT('',(-18.5210615995951,0.,-3.1));
#35225=CARTESIAN_POINT('',(-18.2,0.,-3.1));
#35226=CARTESIAN_POINT('',(-20.,0.,-4.57893840040487));
#35227=CARTESIAN_POINT('',(-20.,0.,-4.57893840040487));
#35228=CARTESIAN_POINT('',(-20.,0.,-9.5));
#35229=CARTESIAN_POINT('',(-20.,0.,-9.5));
#35230=CARTESIAN_POINT('',(-19.5,0.,-10.));
#35231=CARTESIAN_POINT('Origin',(-19.5,0.,-9.49999999999999));
#35232=CARTESIAN_POINT('',(-14.5789384004049,0.,-10.));
#35233=CARTESIAN_POINT('',(-14.5789384004049,0.,-10.));
#35234=CARTESIAN_POINT('',(-13.1,0.,-8.52106159959513));
#35235=CARTESIAN_POINT('',(-14.5789384004049,0.,-10.));
#35236=CARTESIAN_POINT('',(-13.1,0.,-8.2));
#35237=CARTESIAN_POINT('',(-13.1,0.,-8.2));
#35238=CARTESIAN_POINT('',(-15.509308298299,0.,-8.2));
#35239=CARTESIAN_POINT('',(-15.509308298299,0.,-8.2));
#35240=CARTESIAN_POINT('',(-15.509308298299,0.,-6.57452478769713));
#35241=CARTESIAN_POINT('',(-15.509308298299,0.,-8.2));
#35242=CARTESIAN_POINT('',(-12.8347835106019,0.,-3.9));
#35243=CARTESIAN_POINT('',(-15.509308298299,0.,-6.57452478769713));
#35244=CARTESIAN_POINT('',(-7.16521648939811,0.,-3.9));
#35245=CARTESIAN_POINT('',(-6.1,0.,-3.9));
#35246=CARTESIAN_POINT('',(-4.49069170170098,0.,-6.57452478769712));
#35247=CARTESIAN_POINT('',(-4.49069170170098,0.,-6.57452478769712));
#35248=CARTESIAN_POINT('',(-4.49069170170098,0.,-8.19999999999999));
#35249=CARTESIAN_POINT('',(-4.49069170170098,0.,-8.19999999999999));
#35250=CARTESIAN_POINT('',(-6.9,0.,-8.2));
#35251=CARTESIAN_POINT('',(-4.49069170170098,0.,-8.19999999999999));
#35252=CARTESIAN_POINT('',(-6.9,0.,-8.52106159959513));
#35253=CARTESIAN_POINT('',(-6.9,0.,-8.2));
#35254=CARTESIAN_POINT('',(-5.42106159959513,0.,-9.99999999999999));
#35255=CARTESIAN_POINT('',(-6.1,0.,-2.83478351060189));
#35256=CARTESIAN_POINT('',(-3.42547521230287,0.,-5.50930829829901));
#35257=CARTESIAN_POINT('',(-6.1,0.,2.83478351060189));
#35258=CARTESIAN_POINT('',(-6.1,0.,3.9));
#35259=CARTESIAN_POINT('',(-2.69069170170098,0.,6.24409180890091));
#35260=CARTESIAN_POINT('',(-3.42547521230288,0.,5.50930829829902));
#35261=CARTESIAN_POINT('',(-2.69069170170098,0.,8.2));
#35262=CARTESIAN_POINT('',(-2.69069170170098,0.,-0.0866499732000181));
#35263=CARTESIAN_POINT('',(-3.13664997320002,0.,8.2));
#35264=CARTESIAN_POINT('',(-12.1,0.,2.57175827820944E-16));
#35265=CARTESIAN_POINT('Origin',(-10.,0.,0.));
#35266=CARTESIAN_POINT('Origin',(-2.69069170170098,0.,8.2));
#35267=CARTESIAN_POINT('',(-2.69069170170098,500.,8.2));
#35268=CARTESIAN_POINT('',(-2.69069170170098,0.,8.2));
#35269=CARTESIAN_POINT('',(-3.13664997320002,500.,8.2));
#35270=CARTESIAN_POINT('Origin',(-2.69069170170098,0.,6.24409180890091));
#35271=CARTESIAN_POINT('',(-2.69069170170098,500.,6.24409180890091));
#35272=CARTESIAN_POINT('',(-2.69069170170098,0.,6.24409180890091));
#35273=CARTESIAN_POINT('',(-2.69069170170098,500.,-0.0866499732000181));
#35274=CARTESIAN_POINT('Origin',(-6.1,0.,3.9));
#35275=CARTESIAN_POINT('',(-6.1,500.,-2.83478351060189));
#35276=CARTESIAN_POINT('',(-6.1,0.,-2.83478351060189));
#35277=CARTESIAN_POINT('',(-6.1,500.,2.83478351060189));
#35278=CARTESIAN_POINT('',(-6.1,500.,-1.25869587765047));
#35279=CARTESIAN_POINT('',(-6.1,0.,2.83478351060189));
#35280=CARTESIAN_POINT('Origin',(-13.9,0.,3.9));
#35281=CARTESIAN_POINT('',(-12.8347835106019,500.,3.9));
#35282=CARTESIAN_POINT('',(-12.8347835106019,0.,3.9));
#35283=CARTESIAN_POINT('',(-7.16521648939811,500.,3.9));
#35284=CARTESIAN_POINT('',(-7.16521648939811,0.,3.9));
#35285=CARTESIAN_POINT('',(-8.74130412234953,500.,3.9));
#35286=CARTESIAN_POINT('Origin',(-13.9,0.,-3.9));
#35287=CARTESIAN_POINT('',(-13.9,500.,2.83478351060189));
#35288=CARTESIAN_POINT('',(-13.9,0.,2.83478351060189));
#35289=CARTESIAN_POINT('',(-13.9,500.,-2.83478351060189));
#35290=CARTESIAN_POINT('',(-13.9,500.,-5.15869587765047));
#35291=CARTESIAN_POINT('',(-13.9,0.,-2.83478351060189));
#35292=CARTESIAN_POINT('Origin',(-10.,0.,0.));
#35293=CARTESIAN_POINT('',(-12.1,500.,-2.57175827820944E-16));
#35294=CARTESIAN_POINT('',(-12.1,0.,2.57175827820944E-16));
#35295=CARTESIAN_POINT('Origin',(-10.,500.,0.));
#35296=CARTESIAN_POINT('Origin',(-6.1,0.,-3.9));
#35297=CARTESIAN_POINT('',(-7.16521648939811,500.,-3.9));
#35298=CARTESIAN_POINT('',(-7.16521648939811,0.,-3.9));
#35299=CARTESIAN_POINT('',(-12.8347835106019,500.,-3.9));
#35300=CARTESIAN_POINT('',(-12.8347835106019,0.,-3.9));
#35301=CARTESIAN_POINT('',(-4.84130412234953,500.,-3.9));
#35302=CARTESIAN_POINT('Origin',(-15.509308298299,0.,-6.57452478769713));
#35303=CARTESIAN_POINT('',(-15.509308298299,500.,-8.2));
#35304=CARTESIAN_POINT('',(-15.509308298299,0.,-8.2));
#35305=CARTESIAN_POINT('',(-15.509308298299,500.,-6.57452478769713));
#35306=CARTESIAN_POINT('',(-15.509308298299,500.,-6.49595827149903));
#35307=CARTESIAN_POINT('',(-15.509308298299,0.,-6.57452478769713));
#35308=CARTESIAN_POINT('Origin',(-12.8347835106019,0.,-3.9));
#35309=CARTESIAN_POINT('',(-11.1510876329514,500.,-2.21630412234953));
#35310=CARTESIAN_POINT('Origin',(-16.5745247876971,0.,-5.50930829829902));
#35311=CARTESIAN_POINT('',(-16.5745247876971,500.,-5.50930829829902));
#35312=CARTESIAN_POINT('',(-13.5535665161981,500.,-2.48835002679998));
#35313=CARTESIAN_POINT('',(-16.5745247876971,0.,-5.50930829829902));
#35314=CARTESIAN_POINT('Origin',(-18.2,0.,-5.50930829829902));
#35315=CARTESIAN_POINT('',(-18.2,500.,-5.50930829829902));
#35316=CARTESIAN_POINT('',(-10.8913041223495,500.,-5.50930829829901));
#35317=CARTESIAN_POINT('',(-18.2,0.,-5.50930829829902));
#35318=CARTESIAN_POINT('Origin',(-18.2,0.,-3.1));
#35319=CARTESIAN_POINT('',(-18.2,500.,-3.1));
#35320=CARTESIAN_POINT('',(-18.2,500.,-4.75869587765048));
#35321=CARTESIAN_POINT('',(-18.2,0.,-3.1));
#35322=CARTESIAN_POINT('Origin',(-18.5210615995951,0.,-3.1));
#35323=CARTESIAN_POINT('',(-18.5210615995951,500.,-3.1));
#35324=CARTESIAN_POINT('',(-11.0518349221471,500.,-3.1));
#35325=CARTESIAN_POINT('',(-18.5210615995951,0.,-3.1));
#35326=CARTESIAN_POINT('Origin',(-20.,0.,-4.57893840040487));
#35327=CARTESIAN_POINT('',(-20.,500.,-4.57893840040487));
#35328=CARTESIAN_POINT('',(-16.3552653998988,500.,-0.934203800303655));
#35329=CARTESIAN_POINT('',(-20.,0.,-4.57893840040487));
#35330=CARTESIAN_POINT('Origin',(-20.,0.,-9.5));
#35331=CARTESIAN_POINT('',(-20.,500.,-9.5));
#35332=CARTESIAN_POINT('',(-20.,500.,-7.95869587765048));
#35333=CARTESIAN_POINT('',(-20.,0.,-9.5));
#35334=CARTESIAN_POINT('Origin',(-19.5,0.,-9.49999999999999));
#35335=CARTESIAN_POINT('',(-19.5,500.,-10.));
#35336=CARTESIAN_POINT('Origin',(-19.5,500.,-9.49999999999999));
#35337=CARTESIAN_POINT('',(-19.5,0.,-10.));
#35338=CARTESIAN_POINT('Origin',(-14.5789384004049,0.,-10.));
#35339=CARTESIAN_POINT('',(-14.5789384004049,500.,-10.));
#35340=CARTESIAN_POINT('',(-9.08077332255196,500.,-9.99999999999999));
#35341=CARTESIAN_POINT('',(-14.5789384004049,0.,-10.));
#35342=CARTESIAN_POINT('Origin',(-13.1,0.,-8.52106159959513));
#35343=CARTESIAN_POINT('',(-13.1,500.,-8.52106159959513));
#35344=CARTESIAN_POINT('',(-10.1947346001012,500.,-5.61579619969635));
#35345=CARTESIAN_POINT('',(-13.1,0.,-8.52106159959513));
#35346=CARTESIAN_POINT('Origin',(-13.1,0.,-8.2));
#35347=CARTESIAN_POINT('',(-13.1,500.,-8.2));
#35348=CARTESIAN_POINT('',(-13.1,500.,-7.30869587765047));
#35349=CARTESIAN_POINT('',(-13.1,0.,-8.2));
#35350=CARTESIAN_POINT('Origin',(-15.509308298299,0.,-8.2));
#35351=CARTESIAN_POINT('',(-9.54595827149904,500.,-8.2));
#35352=CARTESIAN_POINT('Origin',(-4.49069170170099,0.,6.57452478769713));
#35353=CARTESIAN_POINT('',(-4.49069170170099,500.,8.2));
#35354=CARTESIAN_POINT('',(-4.49069170170099,0.,8.2));
#35355=CARTESIAN_POINT('',(-4.49069170170099,500.,6.57452478769713));
#35356=CARTESIAN_POINT('',(-4.49069170170098,500.,0.0785665161980925));
#35357=CARTESIAN_POINT('',(-4.49069170170099,0.,6.57452478769713));
#35358=CARTESIAN_POINT('Origin',(-7.16521648939811,0.,3.9));
#35359=CARTESIAN_POINT('',(-8.84891236704858,500.,2.21630412234953));
#35360=CARTESIAN_POINT('Origin',(-3.42547521230288,0.,5.50930829829902));
#35361=CARTESIAN_POINT('',(-6.44643348380191,500.,2.48835002679998));
#35362=CARTESIAN_POINT('Origin',(-5.42106159959513,0.,10.));
#35363=CARTESIAN_POINT('',(-5.42106159959513,500.,10.));
#35364=CARTESIAN_POINT('',(-4.5018349221471,500.,10.));
#35365=CARTESIAN_POINT('',(-5.42106159959513,0.,10.));
#35366=CARTESIAN_POINT('Origin',(-6.9,0.,8.52106159959513));
#35367=CARTESIAN_POINT('',(-6.9,500.,8.52106159959513));
#35368=CARTESIAN_POINT('',(-9.80526539989878,500.,5.61579619969636));
#35369=CARTESIAN_POINT('',(-6.9,0.,8.52106159959513));
#35370=CARTESIAN_POINT('Origin',(-6.9,0.,8.2));
#35371=CARTESIAN_POINT('',(-6.9,500.,8.2));
#35372=CARTESIAN_POINT('',(-6.9,500.,0.891304122349527));
#35373=CARTESIAN_POINT('',(-6.9,0.,8.2));
#35374=CARTESIAN_POINT('Origin',(-4.49069170170099,0.,8.2));
#35375=CARTESIAN_POINT('',(-4.03664997320002,500.,8.2));
#35376=CARTESIAN_POINT('Origin',(-16.5745247876971,0.,5.50930829829901));
#35377=CARTESIAN_POINT('',(-18.2,500.,5.50930829829901));
#35378=CARTESIAN_POINT('',(-18.2,0.,5.50930829829901));
#35379=CARTESIAN_POINT('',(-16.5745247876971,500.,5.50930829829901));
#35380=CARTESIAN_POINT('',(-10.0785665161981,500.,5.50930829829901));
#35381=CARTESIAN_POINT('',(-16.5745247876971,0.,5.50930829829901));
#35382=CARTESIAN_POINT('Origin',(-13.9,0.,2.83478351060189));
#35383=CARTESIAN_POINT('',(-9.00760824469906,500.,-2.05760824469905));
#35384=CARTESIAN_POINT('Origin',(-15.509308298299,0.,6.57452478769712));
#35385=CARTESIAN_POINT('',(-15.509308298299,500.,6.57452478769712));
#35386=CARTESIAN_POINT('',(-9.27965414914951,500.,0.34487063854762));
#35387=CARTESIAN_POINT('',(-15.509308298299,0.,6.57452478769712));
#35388=CARTESIAN_POINT('Origin',(-15.509308298299,0.,8.19999999999999));
#35389=CARTESIAN_POINT('',(-15.509308298299,500.,8.19999999999999));
#35390=CARTESIAN_POINT('',(-15.509308298299,500.,0.891304122349518));
#35391=CARTESIAN_POINT('',(-15.509308298299,0.,8.19999999999999));
#35392=CARTESIAN_POINT('Origin',(-13.1,0.,8.2));
#35393=CARTESIAN_POINT('',(-13.1,500.,8.2));
#35394=CARTESIAN_POINT('',(-8.34130412234954,500.,8.2));
#35395=CARTESIAN_POINT('',(-13.1,0.,8.2));
#35396=CARTESIAN_POINT('Origin',(-13.1,0.,8.52106159959513));
#35397=CARTESIAN_POINT('',(-13.1,500.,8.52106159959513));
#35398=CARTESIAN_POINT('',(-13.1,500.,1.05183492214709));
#35399=CARTESIAN_POINT('',(-13.1,0.,8.52106159959513));
#35400=CARTESIAN_POINT('Origin',(-14.5789384004049,0.,10.));
#35401=CARTESIAN_POINT('',(-14.5789384004049,500.,10.));
#35402=CARTESIAN_POINT('',(-7.72550792265318,500.,3.14656952224831));
#35403=CARTESIAN_POINT('',(-14.5789384004049,0.,10.));
#35404=CARTESIAN_POINT('Origin',(-19.5,0.,9.99999999999999));
#35405=CARTESIAN_POINT('',(-19.5,500.,9.99999999999999));
#35406=CARTESIAN_POINT('',(-11.5413041223495,500.,10.));
#35407=CARTESIAN_POINT('',(-19.5,0.,9.99999999999999));
#35408=CARTESIAN_POINT('Origin',(-19.5,0.,9.49999999999999));
#35409=CARTESIAN_POINT('',(-20.,500.,9.49999999999999));
#35410=CARTESIAN_POINT('Origin',(-19.5,500.,9.49999999999999));
#35411=CARTESIAN_POINT('',(-20.,0.,9.49999999999999));
#35412=CARTESIAN_POINT('Origin',(-20.,0.,4.57893840040487));
#35413=CARTESIAN_POINT('',(-20.,500.,4.57893840040487));
#35414=CARTESIAN_POINT('',(-20.,500.,-0.919226677448038));
#35415=CARTESIAN_POINT('',(-20.,0.,4.57893840040487));
#35416=CARTESIAN_POINT('Origin',(-18.5210615995951,0.,3.1));
#35417=CARTESIAN_POINT('',(-18.5210615995951,500.,3.1));
#35418=CARTESIAN_POINT('',(-12.4071003220459,500.,-3.01396127754926));
#35419=CARTESIAN_POINT('',(-18.5210615995951,0.,3.1));
#35420=CARTESIAN_POINT('Origin',(-18.2,0.,3.1));
#35421=CARTESIAN_POINT('',(-18.2,500.,3.1));
#35422=CARTESIAN_POINT('',(-10.8913041223495,500.,3.1));
#35423=CARTESIAN_POINT('',(-18.2,0.,3.1));
#35424=CARTESIAN_POINT('Origin',(-18.2,0.,5.50930829829901));
#35425=CARTESIAN_POINT('',(-18.2,500.,-0.454041728500963));
#35426=CARTESIAN_POINT('Origin',(-6.1,0.,-2.83478351060189));
#35427=CARTESIAN_POINT('',(-4.575,500.,-4.35978351060189));
#35428=CARTESIAN_POINT('Origin',(-4.49069170170098,0.,-6.57452478769712));
#35429=CARTESIAN_POINT('',(-4.49069170170098,500.,-6.57452478769712));
#35430=CARTESIAN_POINT('',(-4.30295409554955,500.,-6.76226239384856));
#35431=CARTESIAN_POINT('',(-4.49069170170098,0.,-6.57452478769712));
#35432=CARTESIAN_POINT('Origin',(-4.49069170170098,0.,-8.19999999999999));
#35433=CARTESIAN_POINT('',(-4.49069170170098,500.,-8.19999999999999));
#35434=CARTESIAN_POINT('',(-4.49069170170098,500.,-7.30869587765047));
#35435=CARTESIAN_POINT('',(-4.49069170170098,0.,-8.19999999999999));
#35436=CARTESIAN_POINT('Origin',(-6.9,0.,-8.2));
#35437=CARTESIAN_POINT('',(-6.9,500.,-8.2));
#35438=CARTESIAN_POINT('',(-5.24130412234953,500.,-8.19999999999999));
#35439=CARTESIAN_POINT('',(-6.9,0.,-8.2));
#35440=CARTESIAN_POINT('Origin',(-6.9,0.,-8.52106159959513));
#35441=CARTESIAN_POINT('',(-6.9,500.,-8.52106159959513));
#35442=CARTESIAN_POINT('',(-6.9,500.,-7.46922667744804));
#35443=CARTESIAN_POINT('',(-6.9,0.,-8.52106159959513));
#35444=CARTESIAN_POINT('Origin',(-5.42106159959513,0.,-9.99999999999999));
#35445=CARTESIAN_POINT('',(-5.42106159959513,500.,-9.99999999999999));
#35446=CARTESIAN_POINT('',(-5.85710032204587,500.,-9.56396127754925));
#35447=CARTESIAN_POINT('',(-5.42106159959513,0.,-9.99999999999999));
#35448=CARTESIAN_POINT('Origin',(-0.500000000000003,0.,-9.99999999999999));
#35449=CARTESIAN_POINT('',(-2.04130412234953,500.,-9.99999999999999));
#35450=CARTESIAN_POINT('Origin',(-3.58260824469906,500.,-6.41739175530094));
#36436=UNCERTAINTY_MEASURE_WITH_UNIT(LENGTH_MEASURE(0.01),#36461,
'DISTANCE_ACCURACY_VALUE',
'Maximum model space distance between geometric entities at asserted c
onnectivities');
#36444=UNCERTAINTY_MEASURE_WITH_UNIT(LENGTH_MEASURE(0.01),#36461,
'DISTANCE_ACCURACY_VALUE',
'Maximum model space distance between geometric entities at asserted c
onnectivities');
#36452=(
GEOMETRIC_REPRESENTATION_CONTEXT(3)
GLOBAL_UNCERTAINTY_ASSIGNED_CONTEXT((#36436))
GLOBAL_UNIT_ASSIGNED_CONTEXT((#36461,#36463,#36464))
REPRESENTATION_CONTEXT('','3D')
);
#36460=(
GEOMETRIC_REPRESENTATION_CONTEXT(3)
GLOBAL_UNCERTAINTY_ASSIGNED_CONTEXT((#36444))
GLOBAL_UNIT_ASSIGNED_CONTEXT((#36461,#36463,#36464))
REPRESENTATION_CONTEXT('','3D')
);
#36461=(
LENGTH_UNIT()
NAMED_UNIT(*)
SI_UNIT(.MILLI.,.METRE.)
);
#36463=(
NAMED_UNIT(*)
PLANE_ANGLE_UNIT()
SI_UNIT($,.RADIAN.)
);
#36464=(
NAMED_UNIT(*)
SI_UNIT($,.STERADIAN.)
SOLID_ANGLE_UNIT()
);
#36472=SHAPE_DEFINITION_REPRESENTATION(#36492,#36523);
#36492=PRODUCT_DEFINITION_SHAPE('',$,#36539);
#36523=SHAPE_REPRESENTATION('',(#12009),#36452);
#36531=PRODUCT_DEFINITION_CONTEXT('part definition',#36578,'design');
#36539=PRODUCT_DEFINITION('V-Slot 20x40','V-Slot 20x40',#36554,#36531);
#36554=PRODUCT_DEFINITION_FORMATION('',$,#36587);
#36578=APPLICATION_CONTEXT(
'Core Data for Automotive Mechanical Design Process');
#36579=PRODUCT_CONTEXT('part definition',#36578,'mechanical');
#36587=PRODUCT('V-Slot 20x40','V-Slot 20x40',$,(#36579));
#36598=PRESENTATION_STYLE_ASSIGNMENT((#36603));
#36603=SURFACE_STYLE_USAGE(.BOTH.,#36608);
#36608=SURFACE_SIDE_STYLE('',(#36613));
#36613=SURFACE_STYLE_FILL_AREA(#36618);
#36618=FILL_AREA_STYLE('Opaque(245,245,246)',(#36623));
#36623=FILL_AREA_STYLE_COLOUR('Opaque(245,245,246)',#36628);
#36628=COLOUR_RGB('Opaque(245,245,246)', 0.40784314, 0.44705882, 0.49803922);
ENDSEC;
END-ISO-10303-21;
